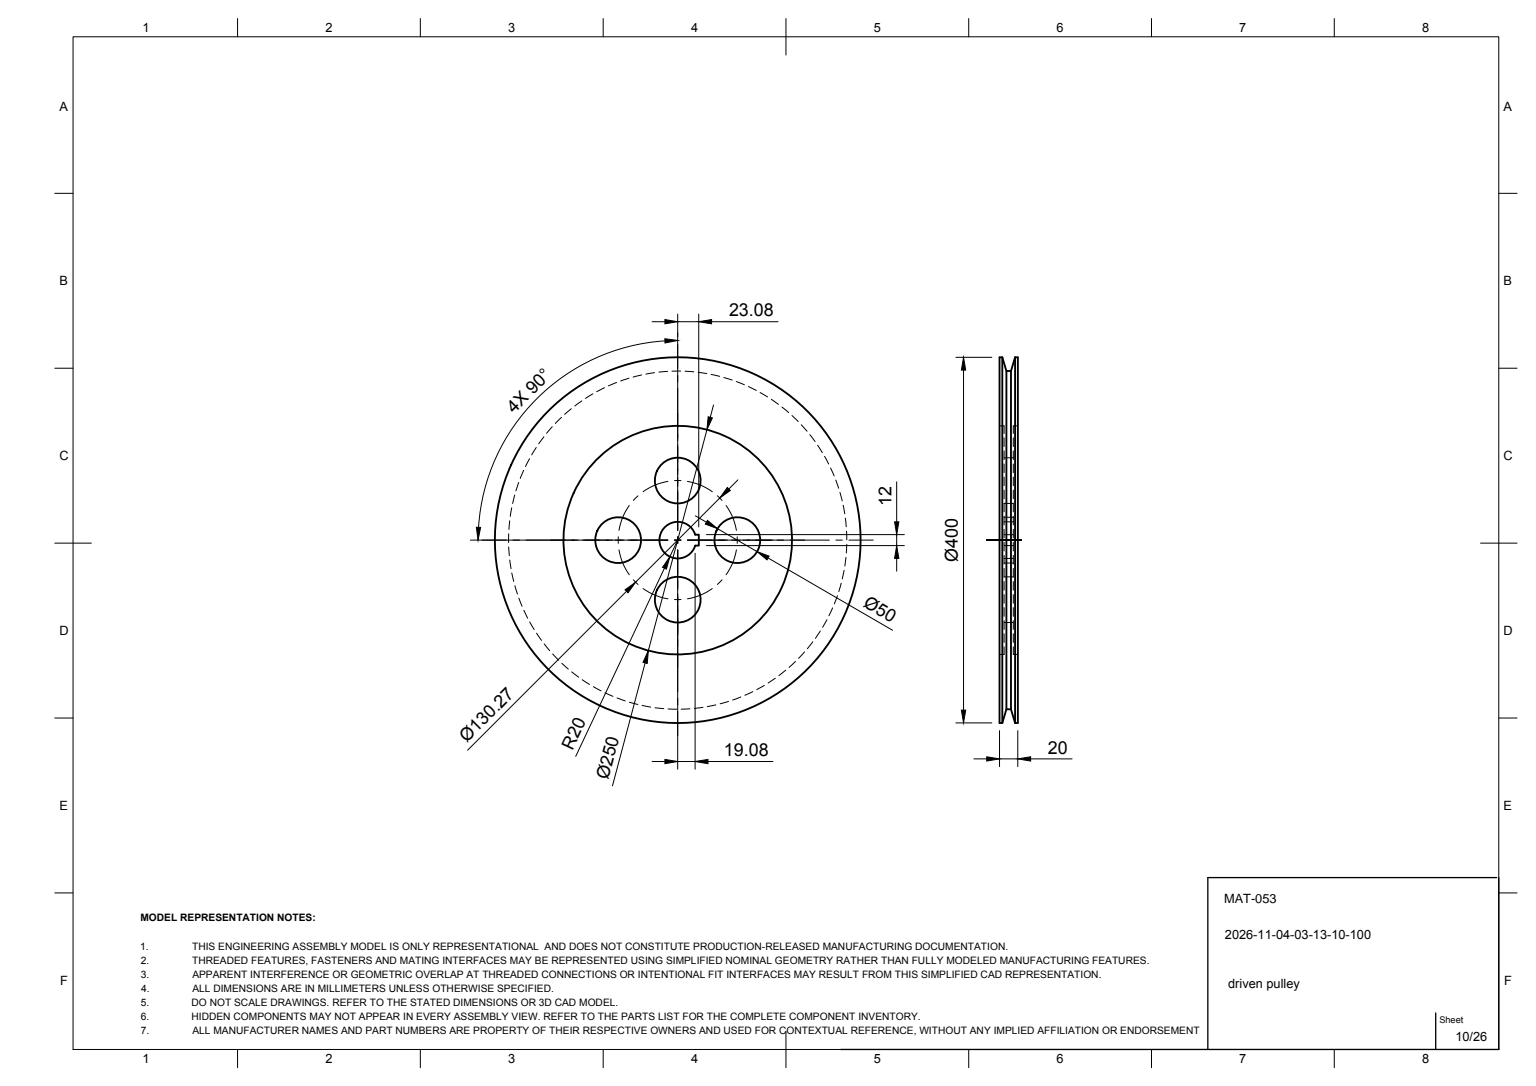
ISO-10303-21;
HEADER;
FILE_DESCRIPTION (('STEP AP214'),
    '1' );
FILE_NAME ('driven pulley.step',
    '2026-10-10T03:43:58',
    ( '' ),
    ( '' ),
    'SwSTEP 2.0',
    'SolidWorks 2026',
    '' );
FILE_SCHEMA (( 'AUTOMOTIVE_DESIGN' ));
ENDSEC;

DATA;
#14=EDGE_CURVE ( 'NONE', #39203, #23906, #5840, .T. ) ;
#73=PRODUCT_DEFINITION_CONTEXT ( 'detailed design', #24706, 'design' ) ;
#203=AXIS2_PLACEMENT_3D ( 'NONE', #23243, #1076, #59454 ) ;
#225=CARTESIAN_POINT ( 'NONE',  ( 90.13282190615606737, 1.839221433318906476E-12, 5.000000000000000000 ) ) ;
#267=CIRCLE ( 'NONE', #18213, 25.00000000000000000 ) ;
#269=ORIENTED_EDGE ( 'NONE', *, *, #50441, .F. ) ;
#325=CARTESIAN_POINT ( 'NONE',  ( 65.13282190615461786, 1.839221433318906476E-12, 5.000000000000000000 ) ) ;
#346=ORIENTED_EDGE ( 'NONE', *, *, #17053, .T. ) ;
#359=CARTESIAN_POINT ( 'NONE',  ( -65.13282190615095146, -1.847197903505587038E-12, 5.000000000000000000 ) ) ;
#383=VERTEX_POINT ( 'NONE', #55130 ) ;
#444=EDGE_LOOP ( 'NONE', ( #35988, #44492, #55517, #13641 ) ) ;
#462=AXIS2_PLACEMENT_3D ( 'NONE', #325, #22133, #54117 ) ;
#539=DIRECTION ( 'NONE',  ( 1.000000000000000000, 0.000000000000000000, 0.000000000000000000 ) ) ;
#586=ORIENTED_EDGE ( 'NONE', *, *, #6995, .F. ) ;
#619=AXIS2_PLACEMENT_3D ( 'NONE', #20593, #9026, #42056 ) ;
#711=CARTESIAN_POINT ( 'NONE',  ( 90.13282190615606737, 1.839221433318906476E-12, -5.000000000000000000 ) ) ;
#800=VECTOR ( 'NONE', #25987, 1000.000000000000000 ) ;
#856=EDGE_CURVE ( 'NONE', #15508, #55490, #4805, .T. ) ;
#868=DIRECTION ( 'NONE',  ( 0.000000000000000000, 1.000000000000000000, 0.000000000000000000 ) ) ;
#1003=VERTEX_POINT ( 'NONE', #17080 ) ;
#1034=DIRECTION ( 'NONE',  ( -1.000000000000000000, 0.000000000000000000, 0.000000000000000000 ) ) ;
#1076=DIRECTION ( 'NONE',  ( 0.000000000000000000, 0.000000000000000000, 1.000000000000000000 ) ) ;
#1234=AXIS2_PLACEMENT_3D ( 'NONE', #59286, #59624, #6531 ) ;
#1238=ORIENTED_EDGE ( 'NONE', *, *, #47800, .F. ) ;
#1338=EDGE_LOOP ( 'NONE', ( #14531, #35591, #15625, #48133 ) ) ;
#1340=CLOSED_SHELL ( 'NONE', ( #64564, #36434, #25846, #2769, #31042, #6717, #35413, #19813, #9481, #33980, #26616, #20112, #10478, #20014, #64798, #13207, #41216, #44725, #21120, #61014, #59716, #10226, #39239, #31844, #27146, #58887, #58375, #11492, #48120, #25762, #35077, #24104 ) ) ;
#1566=EDGE_LOOP ( 'NONE', ( #36926, #54120, #31121, #55593 ) ) ;
#1664=FACE_OUTER_BOUND ( 'NONE', #11943, .T. ) ;
#1697=DIRECTION ( 'NONE',  ( 0.000000000000000000, 0.000000000000000000, -1.000000000000000000 ) ) ;
#1938=VECTOR ( 'NONE', #46028, 1000.000000000000000 ) ;
#1973=DIRECTION ( 'NONE',  ( -0.000000000000000000, -0.000000000000000000, 1.000000000000000000 ) ) ;
#2092=ORIENTED_EDGE ( 'NONE', *, *, #5568, .T. ) ;
#2114=ORIENTED_EDGE ( 'NONE', *, *, #3365, .T. ) ;
#2123=EDGE_LOOP ( 'NONE', ( #65423, #20110, #20744, #32328 ) ) ;
#2127=ORIENTED_EDGE ( 'NONE', *, *, #52497, .F. ) ;
#2164=CARTESIAN_POINT ( 'NONE',  ( 0.000000000000000000, 0.000000000000000000, -5.000000000000000888 ) ) ;
#2182=EDGE_CURVE ( 'NONE', #46584, #55490, #14866, .T. ) ;
#2543=CIRCLE ( 'NONE', #21607, 25.00000000000395772 ) ;
#2575=EDGE_CURVE ( 'NONE', #49581, #11859, #45372, .T. ) ;
#2593=VERTEX_POINT ( 'NONE', #21779 ) ;
#2769=ADVANCED_FACE ( 'NONE', ( #66123 ), #11563, .F. ) ;
#2859=PLANE ( 'NONE',  #68017 ) ;
#3047=FACE_OUTER_BOUND ( 'NONE', #41666, .T. ) ;
#3053=AXIS2_PLACEMENT_3D ( 'NONE', #38989, #1697, #38628 ) ;
#3135=LINE ( 'NONE', #24596, #1938 ) ;
#3146=AXIS2_PLACEMENT_3D ( 'NONE', #50401, #40193, #18044 ) ;
#3280=EDGE_CURVE ( 'NONE', #66579, #13178, #38056, .T. ) ;
#3359=FACE_OUTER_BOUND ( 'NONE', #47238, .T. ) ;
#3365=EDGE_CURVE ( 'NONE', #383, #54841, #53079, .T. ) ;
#3381=DIRECTION ( 'NONE',  ( -0.000000000000000000, -0.000000000000000000, 1.000000000000000000 ) ) ;
#3395=DIRECTION ( 'NONE',  ( 1.000000000000000000, 0.000000000000000000, 0.000000000000000000 ) ) ;
#3412=DIRECTION ( 'NONE',  ( 0.000000000000000000, 0.000000000000000000, 1.000000000000000000 ) ) ;
#3472=SURFACE_SIDE_STYLE ('',( #51665 ) ) ;
#3504=DIRECTION ( 'NONE',  ( 1.000000000000000000, 0.000000000000000000, 0.000000000000000000 ) ) ;
#3630=AXIS2_PLACEMENT_3D ( 'NONE', #28129, #66490, #44673 ) ;
#3954=DIRECTION ( 'NONE',  ( 1.000000000000000000, 0.000000000000000000, 0.000000000000000000 ) ) ;
#3977=DIRECTION ( 'NONE',  ( -0.000000000000000000, -0.000000000000000000, 1.000000000000000000 ) ) ;
#4155=CARTESIAN_POINT ( 'NONE',  ( 0.000000000000000000, 65.13282190615278466, -5.000000000000000000 ) ) ;
#4242=CIRCLE ( 'NONE', #3146, 25.00000000000145306 ) ;
#4276=CIRCLE ( 'NONE', #68301, 25.00000000000296296 ) ;
#4368=DIRECTION ( 'NONE',  ( -0.000000000000000000, -0.000000000000000000, 1.000000000000000000 ) ) ;
#4663=CARTESIAN_POINT ( 'NONE',  ( 185.0000000000000000, 0.000000000000000000, 2.499999999999999556 ) ) ;
#4771=CARTESIAN_POINT ( 'NONE',  ( 0.000000000000000000, 0.000000000000000000, -10.00000000000000000 ) ) ;
#4792=AXIS2_PLACEMENT_3D ( 'NONE', #12377, #6038, #23634 ) ;
#4805=LINE ( 'NONE', #59305, #49723 ) ;
#4840=DIRECTION ( 'NONE',  ( 1.000000000000000000, 0.000000000000000000, 0.000000000000000000 ) ) ;
#4980=CIRCLE ( 'NONE', #462, 25.00000000000145306 ) ;
#5059=DIRECTION ( 'NONE',  ( -0.000000000000000000, -0.000000000000000000, 1.000000000000000000 ) ) ;
#5134=ORIENTED_EDGE ( 'NONE', *, *, #19397, .T. ) ;
#5201=DIRECTION ( 'NONE',  ( -0.000000000000000000, -0.000000000000000000, 1.000000000000000000 ) ) ;
#5272=CARTESIAN_POINT ( 'NONE',  ( -185.0000000000000000, 2.265596578422603396E-14, 2.499999999999999556 ) ) ;
#5548=SHAPE_REPRESENTATION ( 'driven pulley', ( #66832 ), #59007 ) ;
#5568=EDGE_CURVE ( 'NONE', #9677, #15508, #53224, .T. ) ;
#5588=LINE ( 'NONE', #59736, #24033 ) ;
#5840=CIRCLE ( 'NONE', #39560, 25.00000000000296296 ) ;
#5861=ORIENTED_EDGE ( 'NONE', *, *, #61188, .F. ) ;
#5890=DIRECTION ( 'NONE',  ( -1.000000000000000000, 0.000000000000000000, 0.000000000000000000 ) ) ;
#5975=CIRCLE ( 'NONE', #56554, 125.0000000000000000 ) ;
#5999=DIRECTION ( 'NONE',  ( 1.000000000000000000, 0.000000000000000000, 0.000000000000000000 ) ) ;
#6038=DIRECTION ( 'NONE',  ( -0.000000000000000000, -0.000000000000000000, 1.000000000000000000 ) ) ;
#6041=DIRECTION ( 'NONE',  ( 0.000000000000000000, 0.000000000000000000, -1.000000000000000000 ) ) ;
#6180=CARTESIAN_POINT ( 'NONE',  ( 0.000000000000000000, 0.000000000000000000, -10.00000000000000000 ) ) ;
#6277=CONICAL_SURFACE ( 'NONE', #41143, 185.0000000000000000, 1.279339532317029793 ) ;
#6321=PRODUCT ( 'driven pulley', 'driven pulley', '', ( #46640 ) ) ;
#6362=FACE_OUTER_BOUND ( 'NONE', #36222, .T. ) ;
#6459=CARTESIAN_POINT ( 'NONE',  ( 0.000000000000000000, 0.000000000000000000, -20.00000000000000000 ) ) ;
#6531=DIRECTION ( 'NONE',  ( 1.000000000000000000, 0.000000000000000000, 0.000000000000000000 ) ) ;
#6603=EDGE_CURVE ( 'NONE', #47682, #48865, #11766, .T. ) ;
#6627=ORIENTED_EDGE ( 'NONE', *, *, #14136, .F. ) ;
#6717=ADVANCED_FACE ( 'NONE', ( #19558 ), #41706, .F. ) ;
#6816=DIRECTION ( 'NONE',  ( -0.000000000000000000, -0.000000000000000000, 1.000000000000000000 ) ) ;
#6995=EDGE_CURVE ( 'NONE', #34341, #41500, #19660, .T. ) ;
#7019=VERTEX_POINT ( 'NONE', #14245 ) ;
#7023=EDGE_CURVE ( 'NONE', #8320, #22148, #29755, .T. ) ;
#7148=ORIENTED_EDGE ( 'NONE', *, *, #62973, .T. ) ;
#7149=VECTOR ( 'NONE', #29398, 1000.000000000000000 ) ;
#7158=CYLINDRICAL_SURFACE ( 'NONE', #45507, 25.00000000000000000 ) ;
#7185=ORIENTED_EDGE ( 'NONE', *, *, #60905, .F. ) ;
#7296=VECTOR ( 'NONE', #42362, 1000.000000000000000 ) ;
#7368=DIRECTION ( 'NONE',  ( -0.000000000000000000, -0.000000000000000000, 1.000000000000000000 ) ) ;
#7395=ORIENTED_EDGE ( 'NONE', *, *, #7023, .F. ) ;
#7432=EDGE_CURVE ( 'NONE', #19424, #25857, #61573, .T. ) ;
#7456=DIRECTION ( 'NONE',  ( -1.000000000000000000, 0.000000000000000000, 0.000000000000000000 ) ) ;
#7631=CARTESIAN_POINT ( 'NONE',  ( 200.0000000000000000, 2.449293598294706434E-14, -7.000000000000000000 ) ) ;
#7634=DIRECTION ( 'NONE',  ( 1.000000000000000000, 0.000000000000000000, -0.000000000000000000 ) ) ;
#7683=EDGE_LOOP ( 'NONE', ( #65023, #50621 ) ) ;
#7794=FACE_BOUND ( 'NONE', #49270, .T. ) ;
#7869=VECTOR ( 'NONE', #62960, 1000.000000000000000 ) ;
#7933=CYLINDRICAL_SURFACE ( 'NONE', #11850, 125.0000000000000000 ) ;
#7935=EDGE_CURVE ( 'NONE', #49581, #14060, #22990, .T. ) ;
#8124=CARTESIAN_POINT ( 'NONE',  ( 200.0000000000000000, 0.000000000000000000, -10.00000000000000000 ) ) ;
#8137=FACE_BOUND ( 'NONE', #65978, .T. ) ;
#8319=DIRECTION ( 'NONE',  ( 1.000000000000000000, 0.000000000000000000, 0.000000000000000000 ) ) ;
#8320=VERTEX_POINT ( 'NONE', #26711 ) ;
#8335=FACE_OUTER_BOUND ( 'NONE', #67692, .T. ) ;
#8424=AXIS2_PLACEMENT_3D ( 'NONE', #68725, #57497, #24461 ) ;
#8477=DIRECTION ( 'NONE',  ( 0.000000000000000000, 0.000000000000000000, -1.000000000000000000 ) ) ;
#8506=CARTESIAN_POINT ( 'NONE',  ( 0.000000000000000000, 0.000000000000000000, 5.000000000000000000 ) ) ;
#8766=FILL_AREA_STYLE ('',( #37197 ) ) ;
#8813=AXIS2_PLACEMENT_3D ( 'NONE', #50838, #35359, #24117 ) ;
#8817=FACE_OUTER_BOUND ( 'NONE', #68179, .T. ) ;
#9026=DIRECTION ( 'NONE',  ( -0.000000000000000000, -0.000000000000000000, 1.000000000000000000 ) ) ;
#9120=CIRCLE ( 'NONE', #67522, 200.0000000000000000 ) ;
#9344=ORIENTED_EDGE ( 'NONE', *, *, #14136, .T. ) ;
#9481=ADVANCED_FACE ( 'NONE', ( #55813 ), #57673, .F. ) ;
#9514=ORIENTED_EDGE ( 'NONE', *, *, #18668, .F. ) ;
#9516=CARTESIAN_POINT ( 'NONE',  ( 65.13282190615461786, 1.839221433318906476E-12, -5.000000000000000000 ) ) ;
#9594=DIRECTION ( 'NONE',  ( 1.000000000000000000, 0.000000000000000000, 0.000000000000000000 ) ) ;
#9605=EDGE_CURVE ( 'NONE', #11859, #49581, #63695, .T. ) ;
#9650=ORIENTED_EDGE ( 'NONE', *, *, #43482, .T. ) ;
#9656=DIRECTION ( 'NONE',  ( -0.000000000000000000, -0.000000000000000000, 1.000000000000000000 ) ) ;
#9662=CIRCLE ( 'NONE', #62435, 25.00000000000000000 ) ;
#9677=VERTEX_POINT ( 'NONE', #40367 ) ;
#9720=DIRECTION ( 'NONE',  ( 1.000000000000000000, 0.000000000000000000, 0.000000000000000000 ) ) ;
#9736=ORIENTED_EDGE ( 'NONE', *, *, #9605, .T. ) ;
#9853=VECTOR ( 'NONE', #9873, 1000.000000000000227 ) ;
#9873=DIRECTION ( 'NONE',  ( -0.9578262852211514300, 1.172998894335282758E-16, 0.2873478855663451625 ) ) ;
#9903=ORIENTED_EDGE ( 'NONE', *, *, #60097, .T. ) ;
#9908=CIRCLE ( 'NONE', #8813, 125.0000000000000000 ) ;
#9932=ORIENTED_EDGE ( 'NONE', *, *, #24558, .T. ) ;
#10055=CYLINDRICAL_SURFACE ( 'NONE', #17941, 200.0000000000000000 ) ;
#10121=DIRECTION ( 'NONE',  ( -0.000000000000000000, -0.000000000000000000, 1.000000000000000000 ) ) ;
#10127=VECTOR ( 'NONE', #6816, 1000.000000000000000 ) ;
#10174=LINE ( 'NONE', #15801, #50169 ) ;
#10226=ADVANCED_FACE ( 'NONE', ( #11029 ), #47964, .F. ) ;
#10305=DIRECTION ( 'NONE',  ( 1.000000000000000000, 0.000000000000000000, 0.000000000000000000 ) ) ;
#10478=ADVANCED_FACE ( 'NONE', ( #14503 ), #52136, .T. ) ;
#10651=VECTOR ( 'NONE', #35516, 1000.000000000000000 ) ;
#10757=VECTOR ( 'NONE', #66610, 1000.000000000000000 ) ;
#10776=FACE_OUTER_BOUND ( 'NONE', #60970, .T. ) ;
#10963=DIRECTION ( 'NONE',  ( 1.000000000000000000, 0.000000000000000000, 0.000000000000000000 ) ) ;
#11029=FACE_OUTER_BOUND ( 'NONE', #32271, .T. ) ;
#11237=EDGE_LOOP ( 'NONE', ( #63243, #586 ) ) ;
#11388=ORIENTED_EDGE ( 'NONE', *, *, #22251, .T. ) ;
#11419=CARTESIAN_POINT ( 'NONE',  ( 0.000000000000000000, 0.000000000000000000, 7.000000000000000000 ) ) ;
#11460=DIRECTION ( 'NONE',  ( -0.000000000000000000, -0.000000000000000000, 1.000000000000000000 ) ) ;
#11492=ADVANCED_FACE ( 'NONE', ( #63054 ), #36325, .T. ) ;
#11563=CYLINDRICAL_SURFACE ( 'NONE', #66742, 25.00000000000000000 ) ;
#11570=EDGE_CURVE ( 'NONE', #48842, #30587, #49206, .T. ) ;
#11594=DIRECTION ( 'NONE',  ( 1.000000000000000000, 0.000000000000000000, 0.000000000000000000 ) ) ;
#11613=FACE_OUTER_BOUND ( 'NONE', #444, .T. ) ;
#11727=DIRECTION ( 'NONE',  ( 1.000000000000000000, 0.000000000000000000, 0.000000000000000000 ) ) ;
#11754=DIRECTION ( 'NONE',  ( 0.000000000000000000, 0.000000000000000000, -1.000000000000000000 ) ) ;
#11766=CIRCLE ( 'NONE', #51098, 25.00000000000395772 ) ;
#11847=DIRECTION ( 'NONE',  ( 0.000000000000000000, 0.000000000000000000, 1.000000000000000000 ) ) ;
#11850=AXIS2_PLACEMENT_3D ( 'NONE', #55413, #1973, #39938 ) ;
#11859=VERTEX_POINT ( 'NONE', #41177 ) ;
#11943=EDGE_LOOP ( 'NONE', ( #55108, #57726, #64257, #269 ) ) ;
#12116=UNCERTAINTY_MEASURE_WITH_UNIT (LENGTH_MEASURE( 1.000000000000000082E-05 ), #53269, 'distance_accuracy_value', 'NONE');
#12144=EDGE_CURVE ( 'NONE', #41500, #34341, #36731, .T. ) ;
#12358=CARTESIAN_POINT ( 'NONE',  ( -40.13282190614798850, -1.847197903505587038E-12, -9.999999999999998224 ) ) ;
#12377=CARTESIAN_POINT ( 'NONE',  ( 0.000000000000000000, 0.000000000000000000, -2.500000000000002220 ) ) ;
#12449=LINE ( 'NONE', #22649, #10127 ) ;
#12453=VERTEX_POINT ( 'NONE', #39536 ) ;
#12555=DIRECTION ( 'NONE',  ( 1.000000000000000000, 0.000000000000000000, 0.000000000000000000 ) ) ;
#12588=( GEOMETRIC_REPRESENTATION_CONTEXT ( 3 ) GLOBAL_UNCERTAINTY_ASSIGNED_CONTEXT ( ( #66299 ) ) GLOBAL_UNIT_ASSIGNED_CONTEXT ( ( #52001, #41456, #58642 ) ) REPRESENTATION_CONTEXT ( 'NONE', 'WORKASPACE' ) );
#12731=DIRECTION ( 'NONE',  ( 0.000000000000000000, 0.000000000000000000, -1.000000000000000000 ) ) ;
#12848=CARTESIAN_POINT ( 'NONE',  ( -6.000000000000000000, 23.07878402833891229, -5.000000000000000000 ) ) ;
#12948=AXIS2_PLACEMENT_3D ( 'NONE', #36428, #57883, #43795 ) ;
#13029=AXIS2_PLACEMENT_3D ( 'NONE', #6180, #59296, #49077 ) ;
#13063=EDGE_LOOP ( 'NONE', ( #44716, #16709 ) ) ;
#13178=VERTEX_POINT ( 'NONE', #62526 ) ;
#13207=ADVANCED_FACE ( 'NONE', ( #46681, #13987 ), #13638, .F. ) ;
#13252=ORIENTED_EDGE ( 'NONE', *, *, #49764, .T. ) ;
#13260=EDGE_CURVE ( 'NONE', #46584, #50826, #36135, .T. ) ;
#13273=EDGE_CURVE ( 'NONE', #2593, #1003, #15018, .T. ) ;
#13280=AXIS2_PLACEMENT_3D ( 'NONE', #24520, #61100, #3395 ) ;
#13357=CARTESIAN_POINT ( 'NONE',  ( 3.678442866637813759E-12, -65.13282190615278466, -9.999999999999998224 ) ) ;
#13638=PLANE ( 'NONE',  #57238 ) ;
#13640=EDGE_LOOP ( 'NONE', ( #55151, #346, #49689, #9903 ) ) ;
#13641=ORIENTED_EDGE ( 'NONE', *, *, #27798, .F. ) ;
#13927=AXIS2_PLACEMENT_3D ( 'NONE', #54921, #65496, #7456 ) ;
#13987=FACE_OUTER_BOUND ( 'NONE', #47331, .T. ) ;
#14003=VERTEX_POINT ( 'NONE', #63226 ) ;
#14004=LINE ( 'NONE', #25264, #36379 ) ;
#14006=ORIENTED_EDGE ( 'NONE', *, *, #50811, .F. ) ;
#14029=DIRECTION ( 'NONE',  ( -0.000000000000000000, -0.000000000000000000, 1.000000000000000000 ) ) ;
#14054=CARTESIAN_POINT ( 'NONE',  ( 40.13282190615316836, 1.842283050316774879E-12, -9.999999999999998224 ) ) ;
#14060=VERTEX_POINT ( 'NONE', #225 ) ;
#14136=EDGE_CURVE ( 'NONE', #49232, #40260, #32255, .T. ) ;
#14160=ORIENTED_EDGE ( 'NONE', *, *, #45668, .T. ) ;
#14176=ORIENTED_EDGE ( 'NONE', *, *, #12144, .T. ) ;
#14245=CARTESIAN_POINT ( 'NONE',  ( -125.0000000000000000, 1.530808498934191561E-14, 10.00000000000000000 ) ) ;
#14436=LINE ( 'NONE', #35886, #7869 ) ;
#14503=FACE_OUTER_BOUND ( 'NONE', #42414, .T. ) ;
#14531=ORIENTED_EDGE ( 'NONE', *, *, #48902, .T. ) ;
#14558=EDGE_CURVE ( 'NONE', #22538, #40260, #28097, .T. ) ;
#14562=ORIENTED_EDGE ( 'NONE', *, *, #64384, .T. ) ;
#14594=LINE ( 'NONE', #57510, #7296 ) ;
#14599=DIRECTION ( 'NONE',  ( 1.000000000000000000, 0.000000000000000000, 0.000000000000000000 ) ) ;
#14636=EDGE_CURVE ( 'NONE', #22148, #7019, #12449, .T. ) ;
#14671=CARTESIAN_POINT ( 'NONE',  ( 0.000000000000000000, 0.000000000000000000, -10.00000000000000000 ) ) ;
#14693=CARTESIAN_POINT ( 'NONE',  ( -125.0000000000000000, 1.530808498934191561E-14, 5.000000000000000000 ) ) ;
#14839=FACE_OUTER_BOUND ( 'NONE', #54551, .T. ) ;
#14866=LINE ( 'NONE', #15907, #32968 ) ;
#15018=LINE ( 'NONE', #36481, #51616 ) ;
#15085=VECTOR ( 'NONE', #7368, 1000.000000000000000 ) ;
#15127=VERTEX_POINT ( 'NONE', #54034 ) ;
#15371=AXIS2_PLACEMENT_3D ( 'NONE', #21361, #10121, #4840 ) ;
#15442=AXIS2_PLACEMENT_3D ( 'NONE', #6459, #5059, #17347 ) ;
#15508=VERTEX_POINT ( 'NONE', #34629 ) ;
#15539=CARTESIAN_POINT ( 'NONE',  ( 0.000000000000000000, 0.000000000000000000, 7.000000000000000000 ) ) ;
#15543=CARTESIAN_POINT ( 'NONE',  ( -25.00000000000000000, 65.13282190615278466, -5.000000000000000000 ) ) ;
#15625=ORIENTED_EDGE ( 'NONE', *, *, #55396, .T. ) ;
#15739=VERTEX_POINT ( 'NONE', #15543 ) ;
#15801=CARTESIAN_POINT ( 'NONE',  ( 6.000000000000000000, 0.000000000000000000, 5.000000000000000000 ) ) ;
#15907=CARTESIAN_POINT ( 'NONE',  ( -6.000000000000000000, 23.07878402833891229, 9.999999999999998224 ) ) ;
#15924=EDGE_LOOP ( 'NONE', ( #27771, #58045 ) ) ;
#16004=SHAPE_DEFINITION_REPRESENTATION ( #22614, #5548 ) ;
#16034=VECTOR ( 'NONE', #26129, 1000.000000000000227 ) ;
#16044=ORIENTED_EDGE ( 'NONE', *, *, #22064, .F. ) ;
#16128=DIRECTION ( 'NONE',  ( -0.000000000000000000, -0.000000000000000000, 1.000000000000000000 ) ) ;
#16129=CIRCLE ( 'NONE', #37463, 185.0000000000000000 ) ;
#16199=VERTEX_POINT ( 'NONE', #19533 ) ;
#16296=CARTESIAN_POINT ( 'NONE',  ( 0.000000000000000000, 0.000000000000000000, 2.499999999999999556 ) ) ;
#16353=ORIENTED_EDGE ( 'NONE', *, *, #27798, .T. ) ;
#16367=CIRCLE ( 'NONE', #13029, 200.0000000000000000 ) ;
#16554=CIRCLE ( 'NONE', #34567, 20.00000000000000000 ) ;
#16564=CARTESIAN_POINT ( 'NONE',  ( 6.000000000000000000, 23.07878402833891229, 9.999999999999998224 ) ) ;
#16610=CONICAL_SURFACE ( 'NONE', #40229, 200.0000000000000000, 1.279339532317029793 ) ;
#16709=ORIENTED_EDGE ( 'NONE', *, *, #9605, .F. ) ;
#16880=AXIS2_PLACEMENT_3D ( 'NONE', #67142, #46691, #50938 ) ;
#16906=DIRECTION ( 'NONE',  ( -0.000000000000000000, -0.000000000000000000, -1.000000000000000000 ) ) ;
#16915=CARTESIAN_POINT ( 'NONE',  ( 200.0000000000000000, 0.000000000000000000, -7.000000000000000000 ) ) ;
#17022=SHAPE_REPRESENTATION_RELATIONSHIP ( 'NONE' , 'NONE' ,  #5548, #33268 ) ;
#17053=EDGE_CURVE ( 'NONE', #15739, #2593, #267, .T. ) ;
#17080=CARTESIAN_POINT ( 'NONE',  ( 25.00000000000000000, 65.13282190615278466, 5.000000000000000000 ) ) ;
#17159=CARTESIAN_POINT ( 'NONE',  ( 125.0000000000000000, 1.530808498934191561E-14, -5.000000000000000000 ) ) ;
#17347=DIRECTION ( 'NONE',  ( 1.000000000000000000, 0.000000000000000000, 0.000000000000000000 ) ) ;
#17397=LINE ( 'NONE', #60663, #62487 ) ;
#17536=CIRCLE ( 'NONE', #48948, 200.0000000000000000 ) ;
#17603=FACE_OUTER_BOUND ( 'NONE', #19671, .T. ) ;
#17649=ORIENTED_EDGE ( 'NONE', *, *, #57077, .T. ) ;
#17689=AXIS2_PLACEMENT_3D ( 'NONE', #48586, #6041, #63769 ) ;
#17734=DIRECTION ( 'NONE',  ( 0.000000000000000000, 0.000000000000000000, 1.000000000000000000 ) ) ;
#17736=ORIENTED_EDGE ( 'NONE', *, *, #14636, .T. ) ;
#17922=MANIFOLD_SOLID_BREP ( 'Cut-Extrude4', #1340 ) ;
#17941=AXIS2_PLACEMENT_3D ( 'NONE', #4771, #42409, #9720 ) ;
#18044=DIRECTION ( 'NONE',  ( 1.000000000000000000, 0.000000000000000000, 0.000000000000000000 ) ) ;
#18087=CARTESIAN_POINT ( 'NONE',  ( -20.00000000000000000, 2.449293598294706513E-15, 5.000000000000000000 ) ) ;
#18163=ORIENTED_EDGE ( 'NONE', *, *, #13260, .F. ) ;
#18205=AXIS2_PLACEMENT_3D ( 'NONE', #28227, #39156, #54964 ) ;
#18213=AXIS2_PLACEMENT_3D ( 'NONE', #4155, #20663, #67832 ) ;
#18273=CARTESIAN_POINT ( 'NONE',  ( -185.0000000000000000, 2.265596578422603396E-14, 0.000000000000000000 ) ) ;
#18483=ORIENTED_EDGE ( 'NONE', *, *, #14, .F. ) ;
#18581=DIRECTION ( 'NONE',  ( -1.000000000000000000, 0.000000000000000000, 0.000000000000000000 ) ) ;
#18626=FACE_OUTER_BOUND ( 'NONE', #24803, .T. ) ;
#18668=EDGE_CURVE ( 'NONE', #13178, #61651, #9120, .T. ) ;
#18759=AXIS2_PLACEMENT_3D ( 'NONE', #21403, #16128, #37584 ) ;
#18905=EDGE_CURVE ( 'NONE', #22148, #8320, #60773, .T. ) ;
#19110=EDGE_LOOP ( 'NONE', ( #44365, #56046 ) ) ;
#19149=ORIENTED_EDGE ( 'NONE', *, *, #856, .T. ) ;
#19201=PLANE ( 'NONE',  #59888 ) ;
#19209=CIRCLE ( 'NONE', #1234, 200.0000000000000000 ) ;
#19217=DIRECTION ( 'NONE',  ( -1.000000000000000000, 0.000000000000000000, 0.000000000000000000 ) ) ;
#19225=ORIENTED_EDGE ( 'NONE', *, *, #60905, .T. ) ;
#19352=AXIS2_PLACEMENT_3D ( 'NONE', #39406, #38355, #60854 ) ;
#19397=EDGE_CURVE ( 'NONE', #40260, #19424, #46211, .T. ) ;
#19424=VERTEX_POINT ( 'NONE', #24872 ) ;
#19500=AXIS2_PLACEMENT_3D ( 'NONE', #36849, #46702, #62891 ) ;
#19533=CARTESIAN_POINT ( 'NONE',  ( -200.0000000000000000, 2.449293598294706434E-14, -7.000000000000000000 ) ) ;
#19558=FACE_OUTER_BOUND ( 'NONE', #2123, .T. ) ;
#19571=CYLINDRICAL_SURFACE ( 'NONE', #42294, 125.0000000000000000 ) ;
#19645=PRESENTATION_STYLE_ASSIGNMENT (( #24933 ) ) ;
#19655=AXIS2_PLACEMENT_3D ( 'NONE', #53954, #868, #32190 ) ;
#19660=CIRCLE ( 'NONE', #42097, 125.0000000000000000 ) ;
#19671=EDGE_LOOP ( 'NONE', ( #37736, #47416, #9650, #43541 ) ) ;
#19699=CIRCLE ( 'NONE', #35423, 125.0000000000000000 ) ;
#19813=ADVANCED_FACE ( 'NONE', ( #50398 ), #50045, .F. ) ;
#19817=AXIS2_PLACEMENT_3D ( 'NONE', #58441, #37333, #32071 ) ;
#20009=CARTESIAN_POINT ( 'NONE',  ( 125.0000000000000000, 0.000000000000000000, 5.000000000000000000 ) ) ;
#20014=ADVANCED_FACE ( 'NONE', ( #17603 ), #48533, .T. ) ;
#20076=DIRECTION ( 'NONE',  ( 0.000000000000000000, 0.000000000000000000, -1.000000000000000000 ) ) ;
#20110=ORIENTED_EDGE ( 'NONE', *, *, #35090, .T. ) ;
#20112=ADVANCED_FACE ( 'NONE', ( #11613 ), #55225, .T. ) ;
#20210=ORIENTED_EDGE ( 'NONE', *, *, #67936, .T. ) ;
#20221=DIRECTION ( 'NONE',  ( -0.000000000000000000, -0.000000000000000000, 1.000000000000000000 ) ) ;
#20277=ORIENTED_EDGE ( 'NONE', *, *, #18668, .T. ) ;
#20402=AXIS2_PLACEMENT_3D ( 'NONE', #62507, #3412, #40349 ) ;
#20454=CIRCLE ( 'NONE', #50796, 200.0000000000000000 ) ;
#20459=CYLINDRICAL_SURFACE ( 'NONE', #44391, 125.0000000000000000 ) ;
#20508=DIRECTION ( 'NONE',  ( -0.000000000000000000, -0.000000000000000000, 1.000000000000000000 ) ) ;
#20593=CARTESIAN_POINT ( 'NONE',  ( 0.000000000000000000, 0.000000000000000000, -7.000000000000000000 ) ) ;
#20663=DIRECTION ( 'NONE',  ( 0.000000000000000000, 0.000000000000000000, -1.000000000000000000 ) ) ;
#20681=ORIENTED_EDGE ( 'NONE', *, *, #66289, .T. ) ;
#20744=ORIENTED_EDGE ( 'NONE', *, *, #6603, .T. ) ;
#20831=CARTESIAN_POINT ( 'NONE',  ( 0.000000000000000000, 0.000000000000000000, 0.000000000000000000 ) ) ;
#20906=VECTOR ( 'NONE', #16906, 1000.000000000000000 ) ;
#20924=ORIENTED_EDGE ( 'NONE', *, *, #48453, .T. ) ;
#21120=ADVANCED_FACE ( 'NONE', ( #41765, #62877, #47366, #31221, #46688, #56912 ), #57938, .T. ) ;
#21361=CARTESIAN_POINT ( 'NONE',  ( 0.000000000000000000, 0.000000000000000000, 2.499999999999999556 ) ) ;
#21390=ORIENTED_EDGE ( 'NONE', *, *, #58327, .T. ) ;
#21403=CARTESIAN_POINT ( 'NONE',  ( 0.000000000000000000, 0.000000000000000000, -20.00000000000000000 ) ) ;
#21607=AXIS2_PLACEMENT_3D ( 'NONE', #23866, #66793, #18581 ) ;
#21663=EDGE_CURVE ( 'NONE', #9677, #22538, #57861, .T. ) ;
#21760=DIRECTION ( 'NONE',  ( -0.000000000000000000, 1.000000000000000000, 0.000000000000000000 ) ) ;
#21767=DIRECTION ( 'NONE',  ( -0.000000000000000000, -0.000000000000000000, 1.000000000000000000 ) ) ;
#21779=CARTESIAN_POINT ( 'NONE',  ( 25.00000000000000000, 65.13282190615278466, -5.000000000000000000 ) ) ;
#22006=ORIENTED_EDGE ( 'NONE', *, *, #29771, .F. ) ;
#22064=EDGE_CURVE ( 'NONE', #48865, #47682, #49816, .T. ) ;
#22133=DIRECTION ( 'NONE',  ( 0.000000000000000000, 0.000000000000000000, 1.000000000000000000 ) ) ;
#22135=ORIENTED_EDGE ( 'NONE', *, *, #45668, .F. ) ;
#22148=VERTEX_POINT ( 'NONE', #14693 ) ;
#22169=PLANE ( 'NONE',  #56871 ) ;
#22194=LINE ( 'NONE', #16564, #20906 ) ;
#22251=EDGE_CURVE ( 'NONE', #7019, #15127, #5975, .T. ) ;
#22360=VERTEX_POINT ( 'NONE', #49810 ) ;
#22391=DIRECTION ( 'NONE',  ( 1.000000000000000000, 0.000000000000000000, 0.000000000000000000 ) ) ;
#22538=VERTEX_POINT ( 'NONE', #18087 ) ;
#22614=PRODUCT_DEFINITION_SHAPE ( 'NONE', 'NONE',  #63276 ) ;
#22649=CARTESIAN_POINT ( 'NONE',  ( -125.0000000000000000, 1.530808498934191561E-14, 5.000000000000000000 ) ) ;
#22852=EDGE_CURVE ( 'NONE', #2593, #15739, #39742, .T. ) ;
#22990=LINE ( 'NONE', #44434, #10757 ) ;
#23128=AXIS2_PLACEMENT_3D ( 'NONE', #27817, #28518, #5999 ) ;
#23243=CARTESIAN_POINT ( 'NONE',  ( 0.000000000000000000, 0.000000000000000000, -10.00000000000000000 ) ) ;
#23277=CARTESIAN_POINT ( 'NONE',  ( -6.000000000000000000, 23.07878402833891229, 5.000000000000000000 ) ) ;
#23281=AXIS2_PLACEMENT_3D ( 'NONE', #49898, #60100, #66457 ) ;
#23352=FACE_OUTER_BOUND ( 'NONE', #13640, .T. ) ;
#23463=DIRECTION ( 'NONE',  ( 1.000000000000000000, 0.000000000000000000, 0.000000000000000000 ) ) ;
#23529=EDGE_LOOP ( 'NONE', ( #32810, #33867, #50728, #28320 ) ) ;
#23557=DIRECTION ( 'NONE',  ( -0.000000000000000000, -0.000000000000000000, 1.000000000000000000 ) ) ;
#23613=VERTEX_POINT ( 'NONE', #55185 ) ;
#23634=DIRECTION ( 'NONE',  ( 1.000000000000000000, 0.000000000000000000, 0.000000000000000000 ) ) ;
#23699=EDGE_CURVE ( 'NONE', #383, #66579, #40401, .T. ) ;
#23781=CARTESIAN_POINT ( 'NONE',  ( -185.0000000000000000, 2.357445088358655073E-14, 2.499999999999999556 ) ) ;
#23816=CYLINDRICAL_SURFACE ( 'NONE', #13280, 25.00000000000145306 ) ;
#23828=ORIENTED_EDGE ( 'NONE', *, *, #52622, .T. ) ;
#23866=CARTESIAN_POINT ( 'NONE',  ( 3.678442866637813759E-12, -65.13282190615278466, -5.000000000000000000 ) ) ;
#23906=VERTEX_POINT ( 'NONE', #69540 ) ;
#24033=VECTOR ( 'NONE', #21767, 1000.000000000000000 ) ;
#24104=ADVANCED_FACE ( 'NONE', ( #37446 ), #47656, .F. ) ;
#24117=DIRECTION ( 'NONE',  ( 1.000000000000000000, 0.000000000000000000, 0.000000000000000000 ) ) ;
#24429=ORIENTED_EDGE ( 'NONE', *, *, #38176, .F. ) ;
#24461=DIRECTION ( 'NONE',  ( 1.000000000000000000, 0.000000000000000000, 0.000000000000000000 ) ) ;
#24508=CARTESIAN_POINT ( 'NONE',  ( 0.000000000000000000, 0.000000000000000000, 10.00000000000000000 ) ) ;
#24520=CARTESIAN_POINT ( 'NONE',  ( 65.13282190615461786, 1.839221433318906476E-12, -9.999999999999998224 ) ) ;
#24558=EDGE_CURVE ( 'NONE', #15127, #7019, #19699, .T. ) ;
#24596=CARTESIAN_POINT ( 'NONE',  ( -125.0000000000000000, 0.000000000000000000, -5.000000000000000000 ) ) ;
#24706=APPLICATION_CONTEXT ( 'automotive_design' ) ;
#24755=AXIS2_PLACEMENT_3D ( 'NONE', #33572, #17734, #66622 ) ;
#24803=EDGE_LOOP ( 'NONE', ( #53971, #23828, #40146, #57589 ) ) ;
#24805=EDGE_CURVE ( 'NONE', #34775, #16199, #44397, .T. ) ;
#24817=CYLINDRICAL_SURFACE ( 'NONE', #29795, 25.00000000000145306 ) ;
#24872=CARTESIAN_POINT ( 'NONE',  ( 6.000000000000000000, 19.07878402833891229, 4.999999999999997335 ) ) ;
#24933=SURFACE_STYLE_USAGE ( .BOTH. , #3472 ) ;
#24969=ORIENTED_EDGE ( 'NONE', *, *, #7023, .T. ) ;
#25213=FACE_OUTER_BOUND ( 'NONE', #43198, .T. ) ;
#25215=ORIENTED_EDGE ( 'NONE', *, *, #59128, .T. ) ;
#25255=CYLINDRICAL_SURFACE ( 'NONE', #16880, 25.00000000000296296 ) ;
#25264=CARTESIAN_POINT ( 'NONE',  ( -200.0000000000000000, 2.449293598294706434E-14, -10.00000000000000000 ) ) ;
#25296=ORIENTED_EDGE ( 'NONE', *, *, #29875, .F. ) ;
#25762=ADVANCED_FACE ( 'NONE', ( #27432 ), #22169, .F. ) ;
#25808=LINE ( 'NONE', #69393, #58241 ) ;
#25846=ADVANCED_FACE ( 'NONE', ( #38698 ), #6277, .T. ) ;
#25857=VERTEX_POINT ( 'NONE', #33075 ) ;
#25987=DIRECTION ( 'NONE',  ( 0.000000000000000000, -1.000000000000000000, 0.000000000000000000 ) ) ;
#26076=ORIENTED_EDGE ( 'NONE', *, *, #44634, .F. ) ;
#26129=DIRECTION ( 'NONE',  ( 0.9578262852211514300, 0.000000000000000000, 0.2873478855663451625 ) ) ;
#26151=ORIENTED_EDGE ( 'NONE', *, *, #17053, .F. ) ;
#26153=CARTESIAN_POINT ( 'NONE',  ( 0.000000000000000000, 0.000000000000000000, 5.000000000000000000 ) ) ;
#26405=CARTESIAN_POINT ( 'NONE',  ( -40.13282190614798850, -1.847197903505587038E-12, -5.000000000000000000 ) ) ;
#26437=DIRECTION ( 'NONE',  ( -0.000000000000000000, -0.000000000000000000, -1.000000000000000000 ) ) ;
#26576=VECTOR ( 'NONE', #59651, 1000.000000000000000 ) ;
#26616=ADVANCED_FACE ( 'NONE', ( #14839 ), #20459, .F. ) ;
#26711=CARTESIAN_POINT ( 'NONE',  ( 125.0000000000000000, 0.000000000000000000, 5.000000000000000000 ) ) ;
#26713=VECTOR ( 'NONE', #23557, 1000.000000000000000 ) ;
#26852=DIRECTION ( 'NONE',  ( 1.000000000000000000, 0.000000000000000000, 0.000000000000000000 ) ) ;
#26896=CARTESIAN_POINT ( 'NONE',  ( -65.13282190615095146, -1.847197903505587038E-12, -5.000000000000000000 ) ) ;
#26898=( NAMED_UNIT ( * ) SI_UNIT ( $, .STERADIAN. ) SOLID_ANGLE_UNIT ( ) );
#27043=ORIENTED_EDGE ( 'NONE', *, *, #57077, .F. ) ;
#27146=ADVANCED_FACE ( 'NONE', ( #3359 ), #24817, .F. ) ;
#27213=VERTEX_POINT ( 'NONE', #53934 ) ;
#27225=ORIENTED_EDGE ( 'NONE', *, *, #30249, .F. ) ;
#27227=AXIS2_PLACEMENT_3D ( 'NONE', #50247, #29480, #44620 ) ;
#27297=DIRECTION ( 'NONE',  ( 1.000000000000000000, 0.000000000000000000, 0.000000000000000000 ) ) ;
#27353=EDGE_LOOP ( 'NONE', ( #2114, #20924, #45858, #54114 ) ) ;
#27432=FACE_OUTER_BOUND ( 'NONE', #42884, .T. ) ;
#27653=CARTESIAN_POINT ( 'NONE',  ( 20.00000000000000000, 0.000000000000000000, -20.00000000000000000 ) ) ;
#27751=EDGE_CURVE ( 'NONE', #49232, #9677, #48879, .T. ) ;
#27771=ORIENTED_EDGE ( 'NONE', *, *, #63600, .T. ) ;
#27798=EDGE_CURVE ( 'NONE', #22360, #34775, #29236, .T. ) ;
#27817=CARTESIAN_POINT ( 'NONE',  ( 0.000000000000000000, 0.000000000000000000, 2.499999999999999556 ) ) ;
#27839=DIRECTION ( 'NONE',  ( -0.000000000000000000, -0.000000000000000000, 1.000000000000000000 ) ) ;
#28061=ORIENTED_EDGE ( 'NONE', *, *, #14636, .F. ) ;
#28097=CIRCLE ( 'NONE', #24755, 20.00000000000000000 ) ;
#28129=CARTESIAN_POINT ( 'NONE',  ( -65.13282190615095146, -1.847197903505587038E-12, -5.000000000000000000 ) ) ;
#28227=CARTESIAN_POINT ( 'NONE',  ( 0.000000000000000000, 0.000000000000000000, -20.00000000000000000 ) ) ;
#28320=ORIENTED_EDGE ( 'NONE', *, *, #39557, .F. ) ;
#28335=FACE_OUTER_BOUND ( 'NONE', #45849, .T. ) ;
#28388=CARTESIAN_POINT ( 'NONE',  ( 25.00000000000763478, -65.13282190615278466, 5.000000000000000000 ) ) ;
#28518=DIRECTION ( 'NONE',  ( -0.000000000000000000, -0.000000000000000000, 1.000000000000000000 ) ) ;
#28792=VECTOR ( 'NONE', #14029, 1000.000000000000000 ) ;
#29045=AXIS2_PLACEMENT_3D ( 'NONE', #45000, #34476, #44670 ) ;
#29236=LINE ( 'NONE', #8124, #64633 ) ;
#29257=DIRECTION ( 'NONE',  ( -1.000000000000000000, 0.000000000000000000, 0.000000000000000000 ) ) ;
#29280=VERTEX_POINT ( 'NONE', #37196 ) ;
#29398=DIRECTION ( 'NONE',  ( -0.000000000000000000, -0.000000000000000000, 1.000000000000000000 ) ) ;
#29443=CIRCLE ( 'NONE', #3630, 25.00000000000296296 ) ;
#29480=DIRECTION ( 'NONE',  ( -0.000000000000000000, -0.000000000000000000, 1.000000000000000000 ) ) ;
#29571=DIRECTION ( 'NONE',  ( 0.000000000000000000, 0.000000000000000000, 1.000000000000000000 ) ) ;
#29580=FACE_BOUND ( 'NONE', #54135, .T. ) ;
#29723=DIRECTION ( 'NONE',  ( 1.000000000000000000, 0.000000000000000000, 0.000000000000000000 ) ) ;
#29755=CIRCLE ( 'NONE', #8424, 125.0000000000000000 ) ;
#29771=EDGE_CURVE ( 'NONE', #41500, #30587, #3135, .T. ) ;
#29795=AXIS2_PLACEMENT_3D ( 'NONE', #55510, #20221, #14599 ) ;
#29875=EDGE_CURVE ( 'NONE', #35686, #66579, #34480, .T. ) ;
#29893=DIRECTION ( 'NONE',  ( 0.000000000000000000, 0.000000000000000000, 1.000000000000000000 ) ) ;
#30085=VECTOR ( 'NONE', #35338, 1000.000000000000227 ) ;
#30249=EDGE_CURVE ( 'NONE', #12453, #66690, #67119, .T. ) ;
#30587=VERTEX_POINT ( 'NONE', #34108 ) ;
#30615=CIRCLE ( 'NONE', #27227, 200.0000000000000000 ) ;
#30617=EDGE_LOOP ( 'NONE', ( #51747, #54988, #33780, #63979, #32163, #42594 ) ) ;
#30702=AXIS2_PLACEMENT_3D ( 'NONE', #64951, #11460, #27297 ) ;
#30817=VECTOR ( 'NONE', #539, 1000.000000000000000 ) ;
#30908=DIRECTION ( 'NONE',  ( 1.000000000000000000, 0.000000000000000000, 0.000000000000000000 ) ) ;
#30925=CARTESIAN_POINT ( 'NONE',  ( -6.000000000000000000, 23.07878402833891229, -5.000000000000000000 ) ) ;
#30968=VECTOR ( 'NONE', #51368, 1000.000000000000000 ) ;
#31042=ADVANCED_FACE ( 'NONE', ( #8335 ), #23816, .F. ) ;
#31121=ORIENTED_EDGE ( 'NONE', *, *, #50441, .T. ) ;
#31221=FACE_BOUND ( 'NONE', #33575, .T. ) ;
#31328=DIRECTION ( 'NONE',  ( 1.000000000000000000, 0.000000000000000000, 0.000000000000000000 ) ) ;
#31513=LINE ( 'NONE', #48344, #32489 ) ;
#31698=EDGE_CURVE ( 'NONE', #14003, #64820, #50376, .T. ) ;
#31844=ADVANCED_FACE ( 'NONE', ( #18626 ), #40083, .F. ) ;
#32071=DIRECTION ( 'NONE',  ( -1.000000000000000000, 0.000000000000000000, 0.000000000000000000 ) ) ;
#32163=ORIENTED_EDGE ( 'NONE', *, *, #49764, .F. ) ;
#32190=DIRECTION ( 'NONE',  ( 0.000000000000000000, -0.000000000000000000, 1.000000000000000000 ) ) ;
#32255=LINE ( 'NONE', #27653, #26576 ) ;
#32271=EDGE_LOOP ( 'NONE', ( #49506, #2092, #20210, #39875 ) ) ;
#32328=ORIENTED_EDGE ( 'NONE', *, *, #64810, .F. ) ;
#32489=VECTOR ( 'NONE', #53290, 1000.000000000000000 ) ;
#32810=ORIENTED_EDGE ( 'NONE', *, *, #38176, .T. ) ;
#32890=DIRECTION ( 'NONE',  ( -0.000000000000000000, -0.000000000000000000, 1.000000000000000000 ) ) ;
#32902=AXIS2_PLACEMENT_3D ( 'NONE', #41423, #57600, #36488 ) ;
#32968=VECTOR ( 'NONE', #58131, 1000.000000000000000 ) ;
#33040=CARTESIAN_POINT ( 'NONE',  ( 0.000000000000000000, 65.13282190615278466, -9.999999999999998224 ) ) ;
#33075=CARTESIAN_POINT ( 'NONE',  ( 6.000000000000000000, 19.07878402833891229, -5.000000000000000888 ) ) ;
#33268=ADVANCED_BREP_SHAPE_REPRESENTATION ( '', ( #17922, #66832 ), #59007 ) ;
#33520=EDGE_LOOP ( 'NONE', ( #48650, #60012, #41861, #25296 ) ) ;
#33526=AXIS2_PLACEMENT_3D ( 'NONE', #47898, #27839, #10963 ) ;
#33572=CARTESIAN_POINT ( 'NONE',  ( 0.000000000000000000, 0.000000000000000000, 5.000000000000000000 ) ) ;
#33575=EDGE_LOOP ( 'NONE', ( #16044, #57389 ) ) ;
#33600=ORIENTED_EDGE ( 'NONE', *, *, #62973, .F. ) ;
#33780=ORIENTED_EDGE ( 'NONE', *, *, #27751, .F. ) ;
#33848=CARTESIAN_POINT ( 'NONE',  ( 20.00000000000000000, 0.000000000000000000, -5.000000000000000888 ) ) ;
#33867=ORIENTED_EDGE ( 'NONE', *, *, #48903, .T. ) ;
#33980=ADVANCED_FACE ( 'NONE', ( #53137 ), #64754, .F. ) ;
#34066=VECTOR ( 'NONE', #65480, 1000.000000000000000 ) ;
#34108=CARTESIAN_POINT ( 'NONE',  ( -125.0000000000000000, 0.000000000000000000, -10.00000000000000000 ) ) ;
#34186=VERTEX_POINT ( 'NONE', #42522 ) ;
#34341=VERTEX_POINT ( 'NONE', #17159 ) ;
#34464=ORIENTED_EDGE ( 'NONE', *, *, #18905, .F. ) ;
#34476=DIRECTION ( 'NONE',  ( 0.000000000000000000, 0.000000000000000000, 1.000000000000000000 ) ) ;
#34480=CIRCLE ( 'NONE', #15371, 185.0000000000000000 ) ;
#34498=CARTESIAN_POINT ( 'NONE',  ( 0.000000000000000000, 0.000000000000000000, 10.00000000000000000 ) ) ;
#34567=AXIS2_PLACEMENT_3D ( 'NONE', #8506, #39466, #66567 ) ;
#34629=CARTESIAN_POINT ( 'NONE',  ( -5.999999999999998224, 19.07878402833891229, -5.000000000000000000 ) ) ;
#34775=VERTEX_POINT ( 'NONE', #16915 ) ;
#34925=ORIENTED_EDGE ( 'NONE', *, *, #14558, .T. ) ;
#35077=ADVANCED_FACE ( 'NONE', ( #8817 ), #56645, .F. ) ;
#35090=EDGE_CURVE ( 'NONE', #66690, #47682, #14436, .T. ) ;
#35127=CARTESIAN_POINT ( 'NONE',  ( 185.0000000000000000, 0.000000000000000000, 0.000000000000000000 ) ) ;
#35149=CARTESIAN_POINT ( 'NONE',  ( 6.000000000000000000, 23.07878402833891229, -5.000000000000000000 ) ) ;
#35190=DIRECTION ( 'NONE',  ( -0.000000000000000000, 0.000000000000000000, -1.000000000000000000 ) ) ;
#35338=DIRECTION ( 'NONE',  ( -0.9578262852211514300, 0.000000000000000000, -0.2873478855663451625 ) ) ;
#35359=DIRECTION ( 'NONE',  ( -0.000000000000000000, -0.000000000000000000, 1.000000000000000000 ) ) ;
#35413=ADVANCED_FACE ( 'NONE', ( #51971 ), #25255, .F. ) ;
#35423=AXIS2_PLACEMENT_3D ( 'NONE', #62572, #58647, #30908 ) ;
#35502=LINE ( 'NONE', #35149, #800 ) ;
#35516=DIRECTION ( 'NONE',  ( -0.000000000000000000, -0.000000000000000000, 1.000000000000000000 ) ) ;
#35591=ORIENTED_EDGE ( 'NONE', *, *, #2182, .T. ) ;
#35686=VERTEX_POINT ( 'NONE', #23781 ) ;
#35863=EDGE_LOOP ( 'NONE', ( #14176, #44490, #65810, #22006 ) ) ;
#35886=CARTESIAN_POINT ( 'NONE',  ( -25.00000000000028066, -65.13282190615278466, -9.999999999999998224 ) ) ;
#35988=ORIENTED_EDGE ( 'NONE', *, *, #50811, .T. ) ;
#36085=ORIENTED_EDGE ( 'NONE', *, *, #13260, .T. ) ;
#36117=ORIENTED_EDGE ( 'NONE', *, *, #7935, .F. ) ;
#36135=LINE ( 'NONE', #57594, #57193 ) ;
#36195=LINE ( 'NONE', #30925, #30817 ) ;
#36222=EDGE_LOOP ( 'NONE', ( #43180, #59135, #59263, #44775 ) ) ;
#36232=DIRECTION ( 'NONE',  ( 1.000000000000000000, 0.000000000000000000, -0.000000000000000000 ) ) ;
#36325=CYLINDRICAL_SURFACE ( 'NONE', #53672, 185.0000000000000000 ) ;
#36379=VECTOR ( 'NONE', #52662, 1000.000000000000000 ) ;
#36386=EDGE_CURVE ( 'NONE', #383, #34775, #45243, .T. ) ;
#36428=CARTESIAN_POINT ( 'NONE',  ( 3.678442866637813759E-12, -65.13282190615278466, -9.999999999999998224 ) ) ;
#36434=ADVANCED_FACE ( 'NONE', ( #61762 ), #51574, .T. ) ;
#36458=DIRECTION ( 'NONE',  ( 1.000000000000000000, 0.000000000000000000, 0.000000000000000000 ) ) ;
#36481=CARTESIAN_POINT ( 'NONE',  ( 25.00000000000000000, 65.13282190615278466, -9.999999999999998224 ) ) ;
#36488=DIRECTION ( 'NONE',  ( 1.000000000000000000, 0.000000000000000000, -0.000000000000000000 ) ) ;
#36527=EDGE_LOOP ( 'NONE', ( #33600, #55070 ) ) ;
#36656=DIRECTION ( 'NONE',  ( 0.000000000000000000, 0.000000000000000000, 1.000000000000000000 ) ) ;
#36731=CIRCLE ( 'NONE', #23281, 125.0000000000000000 ) ;
#36794=DIRECTION ( 'NONE',  ( -0.000000000000000000, -0.000000000000000000, -1.000000000000000000 ) ) ;
#36849=CARTESIAN_POINT ( 'NONE',  ( 3.678442866637813759E-12, -65.13282190615278466, 5.000000000000000000 ) ) ;
#36926=ORIENTED_EDGE ( 'NONE', *, *, #36386, .F. ) ;
#36968=DIRECTION ( 'NONE',  ( 0.000000000000000000, 0.000000000000000000, 1.000000000000000000 ) ) ;
#37196=CARTESIAN_POINT ( 'NONE',  ( -200.0000000000000000, 2.449293598294706434E-14, -10.00000000000000000 ) ) ;
#37197=FILL_AREA_STYLE_COLOUR ( '', #66486 ) ;
#37271=MECHANICAL_DESIGN_GEOMETRIC_PRESENTATION_REPRESENTATION('',(#52978),#12588);
#37333=DIRECTION ( 'NONE',  ( 0.000000000000000000, 0.000000000000000000, -1.000000000000000000 ) ) ;
#37446=FACE_OUTER_BOUND ( 'NONE', #1338, .T. ) ;
#37463=AXIS2_PLACEMENT_3D ( 'NONE', #67065, #3977, #57785 ) ;
#37584=DIRECTION ( 'NONE',  ( 1.000000000000000000, 0.000000000000000000, 0.000000000000000000 ) ) ;
#37736=ORIENTED_EDGE ( 'NONE', *, *, #64384, .F. ) ;
#37879=CARTESIAN_POINT ( 'NONE',  ( 20.00000000000000000, 0.000000000000000000, 5.000000000000000000 ) ) ;
#38000=DIRECTION ( 'NONE',  ( 0.000000000000000000, 0.000000000000000000, 1.000000000000000000 ) ) ;
#38056=LINE ( 'NONE', #4663, #16034 ) ;
#38176=EDGE_CURVE ( 'NONE', #64281, #34186, #29443, .T. ) ;
#38209=AXIS2_PLACEMENT_3D ( 'NONE', #16296, #4368, #26852 ) ;
#38340=CARTESIAN_POINT ( 'NONE',  ( 0.000000000000000000, 0.000000000000000000, 2.499999999999999556 ) ) ;
#38346=DIRECTION ( 'NONE',  ( 1.000000000000000000, 0.000000000000000000, 0.000000000000000000 ) ) ;
#38355=DIRECTION ( 'NONE',  ( 0.000000000000000000, 0.000000000000000000, 1.000000000000000000 ) ) ;
#38568=CARTESIAN_POINT ( 'NONE',  ( 0.000000000000000000, 0.000000000000000000, 10.00000000000000000 ) ) ;
#38602=DIRECTION ( 'NONE',  ( -1.000000000000000000, 0.000000000000000000, 0.000000000000000000 ) ) ;
#38628=DIRECTION ( 'NONE',  ( -1.000000000000000000, 0.000000000000000000, 0.000000000000000000 ) ) ;
#38698=FACE_OUTER_BOUND ( 'NONE', #68739, .T. ) ;
#38961=CARTESIAN_POINT ( 'NONE',  ( 125.0000000000000000, 1.530808498934191561E-14, -10.00000000000000000 ) ) ;
#38969=DIRECTION ( 'NONE',  ( 0.000000000000000000, 0.000000000000000000, -1.000000000000000000 ) ) ;
#38989=CARTESIAN_POINT ( 'NONE',  ( 65.13282190615461786, 1.839221433318906476E-12, -5.000000000000000000 ) ) ;
#39156=DIRECTION ( 'NONE',  ( -0.000000000000000000, -0.000000000000000000, 1.000000000000000000 ) ) ;
#39203=VERTEX_POINT ( 'NONE', #44165 ) ;
#39236=CONICAL_SURFACE ( 'NONE', #66219, 200.0000000000000000, 1.279339532317029793 ) ;
#39239=ADVANCED_FACE ( 'NONE', ( #10776 ), #53681, .F. ) ;
#39305=DIRECTION ( 'NONE',  ( 0.000000000000000000, 0.000000000000000000, -1.000000000000000000 ) ) ;
#39365=EDGE_LOOP ( 'NONE', ( #53221, #59036, #34925, #6627 ) ) ;
#39383=CARTESIAN_POINT ( 'NONE',  ( -200.0000000000000000, 2.449293598294706434E-14, -10.00000000000000000 ) ) ;
#39406=CARTESIAN_POINT ( 'NONE',  ( 0.000000000000000000, 0.000000000000000000, -10.00000000000000000 ) ) ;
#39466=DIRECTION ( 'NONE',  ( 0.000000000000000000, 0.000000000000000000, 1.000000000000000000 ) ) ;
#39478=ORIENTED_EDGE ( 'NONE', *, *, #47800, .T. ) ;
#39536=CARTESIAN_POINT ( 'NONE',  ( 25.00000000000763478, -65.13282190615278466, -5.000000000000000000 ) ) ;
#39557=EDGE_CURVE ( 'NONE', #64281, #23906, #54554, .T. ) ;
#39560=AXIS2_PLACEMENT_3D ( 'NONE', #359, #38000, #38346 ) ;
#39728=LINE ( 'NONE', #18273, #26713 ) ;
#39742=CIRCLE ( 'NONE', #13927, 25.00000000000000000 ) ;
#39875=ORIENTED_EDGE ( 'NONE', *, *, #49221, .T. ) ;
#39938=DIRECTION ( 'NONE',  ( 1.000000000000000000, 0.000000000000000000, 0.000000000000000000 ) ) ;
#40083=CYLINDRICAL_SURFACE ( 'NONE', #59344, 25.00000000000395772 ) ;
#40146=ORIENTED_EDGE ( 'NONE', *, *, #64810, .T. ) ;
#40193=DIRECTION ( 'NONE',  ( 0.000000000000000000, 0.000000000000000000, 1.000000000000000000 ) ) ;
#40229=AXIS2_PLACEMENT_3D ( 'NONE', #45428, #12731, #29257 ) ;
#40260=VERTEX_POINT ( 'NONE', #37879 ) ;
#40316=DIRECTION ( 'NONE',  ( 0.9578262852211514300, 1.172998894335282758E-16, -0.2873478855663451625 ) ) ;
#40323=CARTESIAN_POINT ( 'NONE',  ( 0.000000000000000000, 65.13282190615278466, 5.000000000000000000 ) ) ;
#40349=DIRECTION ( 'NONE',  ( 1.000000000000000000, 0.000000000000000000, 0.000000000000000000 ) ) ;
#40367=CARTESIAN_POINT ( 'NONE',  ( -20.00000000000000000, 2.449293598294706513E-15, -5.000000000000000888 ) ) ;
#40401=LINE ( 'NONE', #35127, #15085 ) ;
#40484=CARTESIAN_POINT ( 'NONE',  ( 0.000000000000000000, 0.000000000000000000, -5.000000000000000000 ) ) ;
#40661=DIRECTION ( 'NONE',  ( 0.000000000000000000, 0.000000000000000000, 1.000000000000000000 ) ) ;
#40801=CARTESIAN_POINT ( 'NONE',  ( 6.000000000000000000, 19.07878402833891229, -20.00000000000000000 ) ) ;
#41143=AXIS2_PLACEMENT_3D ( 'NONE', #38340, #59783, #11594 ) ;
#41177=CARTESIAN_POINT ( 'NONE',  ( 40.13282190615316836, 1.842283050316774879E-12, -5.000000000000000000 ) ) ;
#41216=ADVANCED_FACE ( 'NONE', ( #46280, #3047 ), #19201, .T. ) ;
#41423=CARTESIAN_POINT ( 'NONE',  ( 0.000000000000000000, 0.000000000000000000, 5.000000000000000000 ) ) ;
#41456=( NAMED_UNIT ( * ) PLANE_ANGLE_UNIT ( ) SI_UNIT ( $, .RADIAN. ) );
#41500=VERTEX_POINT ( 'NONE', #46900 ) ;
#41666=EDGE_LOOP ( 'NONE', ( #47859, #64047 ) ) ;
#41706=CYLINDRICAL_SURFACE ( 'NONE', #12948, 25.00000000000395772 ) ;
#41765=FACE_BOUND ( 'NONE', #54432, .T. ) ;
#41790=ORIENTED_EDGE ( 'NONE', *, *, #2182, .F. ) ;
#41861=ORIENTED_EDGE ( 'NONE', *, *, #23699, .T. ) ;
#41922=DIRECTION ( 'NONE',  ( -0.000000000000000000, -0.000000000000000000, 1.000000000000000000 ) ) ;
#41925=CARTESIAN_POINT ( 'NONE',  ( 0.000000000000000000, 0.000000000000000000, -10.00000000000000000 ) ) ;
#42056=DIRECTION ( 'NONE',  ( 1.000000000000000000, 0.000000000000000000, 0.000000000000000000 ) ) ;
#42062=FACE_OUTER_BOUND ( 'NONE', #61016, .T. ) ;
#42097=AXIS2_PLACEMENT_3D ( 'NONE', #51187, #9656, #29723 ) ;
#42100=ORIENTED_EDGE ( 'NONE', *, *, #7432, .T. ) ;
#42291=DIRECTION ( 'NONE',  ( -0.000000000000000000, -0.000000000000000000, 1.000000000000000000 ) ) ;
#42294=AXIS2_PLACEMENT_3D ( 'NONE', #45958, #36794, #19217 ) ;
#42362=DIRECTION ( 'NONE',  ( 0.000000000000000000, 0.000000000000000000, 1.000000000000000000 ) ) ;
#42409=DIRECTION ( 'NONE',  ( 0.000000000000000000, 0.000000000000000000, 1.000000000000000000 ) ) ;
#42414=EDGE_LOOP ( 'NONE', ( #20277, #14562, #52682, #46406 ) ) ;
#42522=CARTESIAN_POINT ( 'NONE',  ( -90.13282190615392153, -1.844136286507718230E-12, -5.000000000000000000 ) ) ;
#42594=ORIENTED_EDGE ( 'NONE', *, *, #55396, .F. ) ;
#42657=ORIENTED_EDGE ( 'NONE', *, *, #14558, .F. ) ;
#42660=CARTESIAN_POINT ( 'NONE',  ( -185.0000000000000000, 2.265596578422603396E-14, -2.500000000000002220 ) ) ;
#42690=AXIS2_PLACEMENT_3D ( 'NONE', #62264, #36232, #35190 ) ;
#42884=EDGE_LOOP ( 'NONE', ( #36085, #44147, #19149, #41790 ) ) ;
#42994=ORIENTED_EDGE ( 'NONE', *, *, #18905, .T. ) ;
#43059=ORIENTED_EDGE ( 'NONE', *, *, #2575, .T. ) ;
#43062=( NAMED_UNIT ( * ) PLANE_ANGLE_UNIT ( ) SI_UNIT ( $, .RADIAN. ) );
#43180=ORIENTED_EDGE ( 'NONE', *, *, #47563, .F. ) ;
#43198=EDGE_LOOP ( 'NONE', ( #5861, #65959, #67196, #65125 ) ) ;
#43482=EDGE_CURVE ( 'NONE', #13178, #64820, #14594, .T. ) ;
#43509=LINE ( 'NONE', #53716, #59904 ) ;
#43541=ORIENTED_EDGE ( 'NONE', *, *, #31698, .F. ) ;
#43794=CARTESIAN_POINT ( 'NONE',  ( -5.999999999999998224, 19.07878402833891229, 4.999999999999997335 ) ) ;
#43795=DIRECTION ( 'NONE',  ( 1.000000000000000000, 0.000000000000000000, 0.000000000000000000 ) ) ;
#44147=ORIENTED_EDGE ( 'NONE', *, *, #67936, .F. ) ;
#44165=CARTESIAN_POINT ( 'NONE',  ( -90.13282190615392153, -1.844136286507718230E-12, 5.000000000000000000 ) ) ;
#44365=ORIENTED_EDGE ( 'NONE', *, *, #60097, .F. ) ;
#44391=AXIS2_PLACEMENT_3D ( 'NONE', #68647, #41922, #52132 ) ;
#44397=CIRCLE ( 'NONE', #619, 200.0000000000000000 ) ;
#44434=CARTESIAN_POINT ( 'NONE',  ( 90.13282190615606737, 1.839221433318906476E-12, -9.999999999999998224 ) ) ;
#44490=ORIENTED_EDGE ( 'NONE', *, *, #61188, .T. ) ;
#44492=ORIENTED_EDGE ( 'NONE', *, *, #68141, .T. ) ;
#44558=DIRECTION ( 'NONE',  ( 0.000000000000000000, 0.000000000000000000, 1.000000000000000000 ) ) ;
#44620=DIRECTION ( 'NONE',  ( 1.000000000000000000, 0.000000000000000000, 0.000000000000000000 ) ) ;
#44634=EDGE_CURVE ( 'NONE', #29280, #22360, #16367, .T. ) ;
#44670=DIRECTION ( 'NONE',  ( 1.000000000000000000, 0.000000000000000000, 0.000000000000000000 ) ) ;
#44673=DIRECTION ( 'NONE',  ( -1.000000000000000000, 0.000000000000000000, 0.000000000000000000 ) ) ;
#44716=ORIENTED_EDGE ( 'NONE', *, *, #2575, .F. ) ;
#44725=ADVANCED_FACE ( 'NONE', ( #28335 ), #7933, .F. ) ;
#44738=ORIENTED_EDGE ( 'NONE', *, *, #7935, .T. ) ;
#44759=ORIENTED_EDGE ( 'NONE', *, *, #39557, .T. ) ;
#44775=ORIENTED_EDGE ( 'NONE', *, *, #58138, .F. ) ;
#45000=CARTESIAN_POINT ( 'NONE',  ( 0.000000000000000000, 0.000000000000000000, 10.00000000000000000 ) ) ;
#45079=EDGE_CURVE ( 'NONE', #56426, #1003, #67012, .T. ) ;
#45221=ORIENTED_EDGE ( 'NONE', *, *, #7432, .F. ) ;
#45243=LINE ( 'NONE', #7631, #50634 ) ;
#45372=CIRCLE ( 'NONE', #63351, 25.00000000000145306 ) ;
#45428=CARTESIAN_POINT ( 'NONE',  ( 0.000000000000000000, 0.000000000000000000, -7.000000000000000000 ) ) ;
#45507=AXIS2_PLACEMENT_3D ( 'NONE', #50067, #65202, #11727 ) ;
#45550=AXIS2_PLACEMENT_3D ( 'NONE', #2164, #8477, #67917 ) ;
#45668=EDGE_CURVE ( 'NONE', #19424, #27213, #10174, .T. ) ;
#45707=DIRECTION ( 'NONE',  ( 1.000000000000000000, 0.000000000000000000, 0.000000000000000000 ) ) ;
#45849=EDGE_LOOP ( 'NONE', ( #28061, #7395, #19225, #9932 ) ) ;
#45858=ORIENTED_EDGE ( 'NONE', *, *, #66289, .F. ) ;
#45958=CARTESIAN_POINT ( 'NONE',  ( 0.000000000000000000, 0.000000000000000000, -5.000000000000000000 ) ) ;
#46028=DIRECTION ( 'NONE',  ( -0.000000000000000000, -0.000000000000000000, -1.000000000000000000 ) ) ;
#46211=CIRCLE ( 'NONE', #20402, 20.00000000000000000 ) ;
#46240=ORIENTED_EDGE ( 'NONE', *, *, #48903, .F. ) ;
#46280=FACE_BOUND ( 'NONE', #7683, .T. ) ;
#46311=CARTESIAN_POINT ( 'NONE',  ( -65.13282190615095146, -1.847197903505587038E-12, 5.000000000000000000 ) ) ;
#46406=ORIENTED_EDGE ( 'NONE', *, *, #43482, .F. ) ;
#46584=VERTEX_POINT ( 'NONE', #23277 ) ;
#46638=ORIENTED_EDGE ( 'NONE', *, *, #56377, .F. ) ;
#46640=PRODUCT_CONTEXT ( 'NONE', #48895, 'mechanical' ) ;
#46681=FACE_BOUND ( 'NONE', #15924, .T. ) ;
#46688=FACE_BOUND ( 'NONE', #68032, .T. ) ;
#46691=DIRECTION ( 'NONE',  ( -0.000000000000000000, -0.000000000000000000, 1.000000000000000000 ) ) ;
#46702=DIRECTION ( 'NONE',  ( 0.000000000000000000, 0.000000000000000000, 1.000000000000000000 ) ) ;
#46900=CARTESIAN_POINT ( 'NONE',  ( -125.0000000000000000, 0.000000000000000000, -5.000000000000000000 ) ) ;
#47238=EDGE_LOOP ( 'NONE', ( #27043, #9736, #44738, #7148 ) ) ;
#47331=EDGE_LOOP ( 'NONE', ( #14006, #26076 ) ) ;
#47366=FACE_BOUND ( 'NONE', #36527, .T. ) ;
#47416=ORIENTED_EDGE ( 'NONE', *, *, #58138, .T. ) ;
#47563=EDGE_CURVE ( 'NONE', #35686, #61651, #53443, .T. ) ;
#47605=AXIS2_PLACEMENT_3D ( 'NONE', #65346, #38969, #5890 ) ;
#47656=PLANE ( 'NONE',  #19655 ) ;
#47682=VERTEX_POINT ( 'NONE', #58722 ) ;
#47800=EDGE_CURVE ( 'NONE', #34186, #64281, #4276, .T. ) ;
#47848=DIRECTION ( 'NONE',  ( -1.000000000000000000, 0.000000000000000000, 0.000000000000000000 ) ) ;
#47859=ORIENTED_EDGE ( 'NONE', *, *, #66822, .T. ) ;
#47898=CARTESIAN_POINT ( 'NONE',  ( 0.000000000000000000, 0.000000000000000000, -10.00000000000000000 ) ) ;
#47923=CARTESIAN_POINT ( 'NONE',  ( 0.000000000000000000, 23.07878402833891229, 5.000000000000000000 ) ) ;
#47964=CYLINDRICAL_SURFACE ( 'NONE', #15442, 20.00000000000000000 ) ;
#48117=EDGE_LOOP ( 'NONE', ( #24969, #42994 ) ) ;
#48120=ADVANCED_FACE ( 'NONE', ( #56329 ), #16610, .T. ) ;
#48133=ORIENTED_EDGE ( 'NONE', *, *, #58327, .F. ) ;
#48183=CARTESIAN_POINT ( 'NONE',  ( -6.000000000000000000, 23.07878402833891229, 9.999999999999998224 ) ) ;
#48344=CARTESIAN_POINT ( 'NONE',  ( 25.00000000000763478, -65.13282190615278466, -9.999999999999998224 ) ) ;
#48378=DIRECTION ( 'NONE',  ( -0.000000000000000000, 1.000000000000000000, -0.000000000000000000 ) ) ;
#48447=ORIENTED_EDGE ( 'NONE', *, *, #52622, .F. ) ;
#48453=EDGE_CURVE ( 'NONE', #54841, #35686, #39728, .T. ) ;
#48533=CYLINDRICAL_SURFACE ( 'NONE', #203, 200.0000000000000000 ) ;
#48586=CARTESIAN_POINT ( 'NONE',  ( 3.678442866637813759E-12, -65.13282190615278466, -5.000000000000000000 ) ) ;
#48650=ORIENTED_EDGE ( 'NONE', *, *, #48453, .F. ) ;
#48814=VERTEX_POINT ( 'NONE', #66404 ) ;
#48842=VERTEX_POINT ( 'NONE', #38961 ) ;
#48865=VERTEX_POINT ( 'NONE', #28388 ) ;
#48879=CIRCLE ( 'NONE', #45550, 20.00000000000000000 ) ;
#48895=APPLICATION_CONTEXT ( 'automotive_design' ) ;
#48902=EDGE_CURVE ( 'NONE', #27213, #46584, #63433, .T. ) ;
#48903=EDGE_CURVE ( 'NONE', #34186, #39203, #25808, .T. ) ;
#48948=AXIS2_PLACEMENT_3D ( 'NONE', #15539, #58429, #53140 ) ;
#49077=DIRECTION ( 'NONE',  ( 1.000000000000000000, 0.000000000000000000, 0.000000000000000000 ) ) ;
#49132=CARTESIAN_POINT ( 'NONE',  ( 0.000000000000000000, 0.000000000000000000, -7.000000000000000000 ) ) ;
#49206=CIRCLE ( 'NONE', #33526, 125.0000000000000000 ) ;
#49221=EDGE_CURVE ( 'NONE', #50826, #22538, #16554, .T. ) ;
#49232=VERTEX_POINT ( 'NONE', #33848 ) ;
#49270=EDGE_LOOP ( 'NONE', ( #63317, #26151 ) ) ;
#49506=ORIENTED_EDGE ( 'NONE', *, *, #21663, .F. ) ;
#49567=LINE ( 'NONE', #39383, #56053 ) ;
#49581=VERTEX_POINT ( 'NONE', #711 ) ;
#49601=ORIENTED_EDGE ( 'NONE', *, *, #45079, .T. ) ;
#49689=ORIENTED_EDGE ( 'NONE', *, *, #13273, .T. ) ;
#49723=VECTOR ( 'NONE', #48378, 1000.000000000000000 ) ;
#49764=EDGE_CURVE ( 'NONE', #23613, #25857, #35502, .T. ) ;
#49810=CARTESIAN_POINT ( 'NONE',  ( 200.0000000000000000, 0.000000000000000000, -10.00000000000000000 ) ) ;
#49816=CIRCLE ( 'NONE', #19500, 25.00000000000395772 ) ;
#49898=CARTESIAN_POINT ( 'NONE',  ( 0.000000000000000000, 0.000000000000000000, -5.000000000000000000 ) ) ;
#49925=AXIS2_PLACEMENT_3D ( 'NONE', #46311, #50908, #36458 ) ;
#50045=CYLINDRICAL_SURFACE ( 'NONE', #18205, 20.00000000000000000 ) ;
#50067=CARTESIAN_POINT ( 'NONE',  ( 0.000000000000000000, 65.13282190615278466, -9.999999999999998224 ) ) ;
#50169=VECTOR ( 'NONE', #21760, 1000.000000000000000 ) ;
#50247=CARTESIAN_POINT ( 'NONE',  ( 0.000000000000000000, 0.000000000000000000, -7.000000000000000000 ) ) ;
#50292=AXIS2_PLACEMENT_3D ( 'NONE', #41925, #36656, #3954 ) ;
#50376=CIRCLE ( 'NONE', #29045, 200.0000000000000000 ) ;
#50398=FACE_OUTER_BOUND ( 'NONE', #39365, .T. ) ;
#50401=CARTESIAN_POINT ( 'NONE',  ( 65.13282190615461786, 1.839221433318906476E-12, 5.000000000000000000 ) ) ;
#50441=EDGE_CURVE ( 'NONE', #54841, #16199, #51172, .T. ) ;
#50530=CARTESIAN_POINT ( 'NONE',  ( 0.000000000000000000, 0.000000000000000000, 0.000000000000000000 ) ) ;
#50621=ORIENTED_EDGE ( 'NONE', *, *, #22251, .F. ) ;
#50634=VECTOR ( 'NONE', #40316, 1000.000000000000227 ) ;
#50690=AXIS2_PLACEMENT_3D ( 'NONE', #26153, #69042, #10305 ) ;
#50717=CARTESIAN_POINT ( 'NONE',  ( -200.0000000000000000, 2.449293598294706434E-14, 7.000000000000000000 ) ) ;
#50728=ORIENTED_EDGE ( 'NONE', *, *, #14, .T. ) ;
#50796=AXIS2_PLACEMENT_3D ( 'NONE', #34498, #29893, #3504 ) ;
#50811=EDGE_CURVE ( 'NONE', #22360, #29280, #19209, .T. ) ;
#50826=VERTEX_POINT ( 'NONE', #43794 ) ;
#50838=CARTESIAN_POINT ( 'NONE',  ( 0.000000000000000000, 0.000000000000000000, -10.00000000000000000 ) ) ;
#50908=DIRECTION ( 'NONE',  ( 0.000000000000000000, 0.000000000000000000, 1.000000000000000000 ) ) ;
#50938=DIRECTION ( 'NONE',  ( 1.000000000000000000, 0.000000000000000000, 0.000000000000000000 ) ) ;
#51049=FACE_OUTER_BOUND ( 'NONE', #11237, .T. ) ;
#51098=AXIS2_PLACEMENT_3D ( 'NONE', #57200, #51579, #51231 ) ;
#51172=LINE ( 'NONE', #51520, #30085 ) ;
#51187=CARTESIAN_POINT ( 'NONE',  ( 0.000000000000000000, 0.000000000000000000, -5.000000000000000000 ) ) ;
#51231=DIRECTION ( 'NONE',  ( 1.000000000000000000, 0.000000000000000000, 0.000000000000000000 ) ) ;
#51368=DIRECTION ( 'NONE',  ( 0.000000000000000000, 0.000000000000000000, -1.000000000000000000 ) ) ;
#51520=CARTESIAN_POINT ( 'NONE',  ( -200.0000000000000000, 0.000000000000000000, -7.000000000000000000 ) ) ;
#51557=CARTESIAN_POINT ( 'NONE',  ( -20.00000000000000000, 2.449293598294706513E-15, -20.00000000000000000 ) ) ;
#51574=CYLINDRICAL_SURFACE ( 'NONE', #68608, 185.0000000000000000 ) ;
#51579=DIRECTION ( 'NONE',  ( 0.000000000000000000, 0.000000000000000000, 1.000000000000000000 ) ) ;
#51616=VECTOR ( 'NONE', #52645, 1000.000000000000000 ) ;
#51623=DIRECTION ( 'NONE',  ( 0.000000000000000000, 0.000000000000000000, 1.000000000000000000 ) ) ;
#51665=SURFACE_STYLE_FILL_AREA ( #8766 ) ;
#51747=ORIENTED_EDGE ( 'NONE', *, *, #856, .F. ) ;
#51971=FACE_OUTER_BOUND ( 'NONE', #23529, .T. ) ;
#52001=( LENGTH_UNIT ( ) NAMED_UNIT ( * ) SI_UNIT ( .MILLI., .METRE. ) );
#52132=DIRECTION ( 'NONE',  ( 1.000000000000000000, 0.000000000000000000, 0.000000000000000000 ) ) ;
#52136=CYLINDRICAL_SURFACE ( 'NONE', #50292, 200.0000000000000000 ) ;
#52341=PRODUCT_DEFINITION_FORMATION_WITH_SPECIFIED_SOURCE ( 'ANY', '', #6321, .NOT_KNOWN. ) ;
#52424=DIRECTION ( 'NONE',  ( 0.000000000000000000, 0.000000000000000000, -1.000000000000000000 ) ) ;
#52497=EDGE_CURVE ( 'NONE', #16199, #34775, #30615, .T. ) ;
#52614=VECTOR ( 'NONE', #63783, 1000.000000000000000 ) ;
#52622=EDGE_CURVE ( 'NONE', #66690, #12453, #2543, .T. ) ;
#52645=DIRECTION ( 'NONE',  ( -0.000000000000000000, -0.000000000000000000, 1.000000000000000000 ) ) ;
#52662=DIRECTION ( 'NONE',  ( 0.000000000000000000, 0.000000000000000000, 1.000000000000000000 ) ) ;
#52682=ORIENTED_EDGE ( 'NONE', *, *, #66822, .F. ) ;
#52978=STYLED_ITEM ( 'NONE', ( #19645 ), #17922 ) ;
#53001=DIRECTION ( 'NONE',  ( 0.000000000000000000, 0.000000000000000000, 1.000000000000000000 ) ) ;
#53079=CIRCLE ( 'NONE', #4792, 185.0000000000000000 ) ;
#53137=FACE_OUTER_BOUND ( 'NONE', #35863, .T. ) ;
#53140=DIRECTION ( 'NONE',  ( 1.000000000000000000, 0.000000000000000000, 0.000000000000000000 ) ) ;
#53221=ORIENTED_EDGE ( 'NONE', *, *, #27751, .T. ) ;
#53224=CIRCLE ( 'NONE', #47605, 20.00000000000000000 ) ;
#53269=( LENGTH_UNIT ( ) NAMED_UNIT ( * ) SI_UNIT ( .MILLI., .METRE. ) );
#53290=DIRECTION ( 'NONE',  ( -0.000000000000000000, -0.000000000000000000, 1.000000000000000000 ) ) ;
#53443=LINE ( 'NONE', #5272, #9853 ) ;
#53672=AXIS2_PLACEMENT_3D ( 'NONE', #20831, #42291, #9594 ) ;
#53681=CYLINDRICAL_SURFACE ( 'NONE', #30702, 25.00000000000296296 ) ;
#53716=CARTESIAN_POINT ( 'NONE',  ( -25.00000000000000000, 65.13282190615278466, -9.999999999999998224 ) ) ;
#53925=DIRECTION ( 'NONE',  ( 0.000000000000000000, 0.000000000000000000, 1.000000000000000000 ) ) ;
#53934=CARTESIAN_POINT ( 'NONE',  ( 6.000000000000000000, 23.07878402833891229, 5.000000000000000000 ) ) ;
#53954=CARTESIAN_POINT ( 'NONE',  ( -6.000000000000000000, 23.07878402833891229, 9.999999999999998224 ) ) ;
#53971=ORIENTED_EDGE ( 'NONE', *, *, #35090, .F. ) ;
#54034=CARTESIAN_POINT ( 'NONE',  ( 125.0000000000000000, 0.000000000000000000, 10.00000000000000000 ) ) ;
#54101=EDGE_CURVE ( 'NONE', #15739, #56426, #43509, .T. ) ;
#54114=ORIENTED_EDGE ( 'NONE', *, *, #23699, .F. ) ;
#54117=DIRECTION ( 'NONE',  ( 1.000000000000000000, 0.000000000000000000, 0.000000000000000000 ) ) ;
#54120=ORIENTED_EDGE ( 'NONE', *, *, #68379, .F. ) ;
#54135=EDGE_LOOP ( 'NONE', ( #24429, #1238 ) ) ;
#54327=DIRECTION ( 'NONE',  ( 1.000000000000000000, 0.000000000000000000, 0.000000000000000000 ) ) ;
#54432=EDGE_LOOP ( 'NONE', ( #18163, #63492, #22135, #56830, #42657, #67159 ) ) ;
#54551=EDGE_LOOP ( 'NONE', ( #34464, #17736, #11388, #7185 ) ) ;
#54554=LINE ( 'NONE', #12358, #34066 ) ;
#54571=AXIS2_PLACEMENT_3D ( 'NONE', #65199, #53925, #59900 ) ;
#54831=DIRECTION ( 'NONE',  ( 1.000000000000000000, 0.000000000000000000, 0.000000000000000000 ) ) ;
#54841=VERTEX_POINT ( 'NONE', #42660 ) ;
#54921=CARTESIAN_POINT ( 'NONE',  ( 0.000000000000000000, 65.13282190615278466, -5.000000000000000000 ) ) ;
#54923=CIRCLE ( 'NONE', #38209, 185.0000000000000000 ) ;
#54964=DIRECTION ( 'NONE',  ( 1.000000000000000000, 0.000000000000000000, 0.000000000000000000 ) ) ;
#54988=ORIENTED_EDGE ( 'NONE', *, *, #5568, .F. ) ;
#55070=ORIENTED_EDGE ( 'NONE', *, *, #68976, .F. ) ;
#55108=ORIENTED_EDGE ( 'NONE', *, *, #3365, .F. ) ;
#55130=CARTESIAN_POINT ( 'NONE',  ( 185.0000000000000000, 0.000000000000000000, -2.500000000000002220 ) ) ;
#55151=ORIENTED_EDGE ( 'NONE', *, *, #54101, .F. ) ;
#55185=CARTESIAN_POINT ( 'NONE',  ( 6.000000000000000000, 23.07878402833891229, -5.000000000000000000 ) ) ;
#55225=CYLINDRICAL_SURFACE ( 'NONE', #19352, 200.0000000000000000 ) ;
#55396=EDGE_CURVE ( 'NONE', #55490, #23613, #36195, .T. ) ;
#55407=ORIENTED_EDGE ( 'NONE', *, *, #68976, .T. ) ;
#55413=CARTESIAN_POINT ( 'NONE',  ( 0.000000000000000000, 0.000000000000000000, 5.000000000000000000 ) ) ;
#55490=VERTEX_POINT ( 'NONE', #12848 ) ;
#55510=CARTESIAN_POINT ( 'NONE',  ( 65.13282190615461786, 1.839221433318906476E-12, -9.999999999999998224 ) ) ;
#55517=ORIENTED_EDGE ( 'NONE', *, *, #24805, .F. ) ;
#55553=DIRECTION ( 'NONE',  ( 0.000000000000000000, 0.000000000000000000, 1.000000000000000000 ) ) ;
#55554=CIRCLE ( 'NONE', #49925, 25.00000000000296296 ) ;
#55593=ORIENTED_EDGE ( 'NONE', *, *, #52497, .T. ) ;
#55761=CIRCLE ( 'NONE', #19817, 20.00000000000000000 ) ;
#55813=FACE_OUTER_BOUND ( 'NONE', #56384, .T. ) ;
#56046=ORIENTED_EDGE ( 'NONE', *, *, #45079, .F. ) ;
#56053=VECTOR ( 'NONE', #55553, 1000.000000000000000 ) ;
#56124=ORIENTED_EDGE ( 'NONE', *, *, #54101, .T. ) ;
#56252=DIRECTION ( 'NONE',  ( -0.000000000000000000, -0.000000000000000000, 1.000000000000000000 ) ) ;
#56316=FACE_BOUND ( 'NONE', #13063, .T. ) ;
#56329=FACE_OUTER_BOUND ( 'NONE', #1566, .T. ) ;
#56377=EDGE_CURVE ( 'NONE', #23906, #39203, #55554, .T. ) ;
#56384=EDGE_LOOP ( 'NONE', ( #25215, #9344, #5134, #42100 ) ) ;
#56426=VERTEX_POINT ( 'NONE', #69142 ) ;
#56554=AXIS2_PLACEMENT_3D ( 'NONE', #38568, #53001, #22391 ) ;
#56634=ORIENTED_EDGE ( 'NONE', *, *, #68141, .F. ) ;
#56645=PLANE ( 'NONE',  #42690 ) ;
#56830=ORIENTED_EDGE ( 'NONE', *, *, #19397, .F. ) ;
#56871=AXIS2_PLACEMENT_3D ( 'NONE', #48183, #47848, #36968 ) ;
#56912=FACE_OUTER_BOUND ( 'NONE', #48117, .T. ) ;
#57077=EDGE_CURVE ( 'NONE', #11859, #48814, #62239, .T. ) ;
#57193=VECTOR ( 'NONE', #68488, 1000.000000000000000 ) ;
#57200=CARTESIAN_POINT ( 'NONE',  ( 3.678442866637813759E-12, -65.13282190615278466, 5.000000000000000000 ) ) ;
#57238=AXIS2_PLACEMENT_3D ( 'NONE', #14671, #51623, #57245 ) ;
#57245=DIRECTION ( 'NONE',  ( 1.000000000000000000, 0.000000000000000000, -0.000000000000000000 ) ) ;
#57294=LINE ( 'NONE', #20009, #28792 ) ;
#57389=ORIENTED_EDGE ( 'NONE', *, *, #6603, .F. ) ;
#57497=DIRECTION ( 'NONE',  ( 0.000000000000000000, 0.000000000000000000, 1.000000000000000000 ) ) ;
#57510=CARTESIAN_POINT ( 'NONE',  ( 200.0000000000000000, 0.000000000000000000, -10.00000000000000000 ) ) ;
#57589=ORIENTED_EDGE ( 'NONE', *, *, #22064, .T. ) ;
#57594=CARTESIAN_POINT ( 'NONE',  ( -6.000000000000000000, 0.000000000000000000, 5.000000000000000000 ) ) ;
#57600=DIRECTION ( 'NONE',  ( 0.000000000000000000, 0.000000000000000000, 1.000000000000000000 ) ) ;
#57673=CYLINDRICAL_SURFACE ( 'NONE', #18759, 20.00000000000000000 ) ;
#57726=ORIENTED_EDGE ( 'NONE', *, *, #36386, .T. ) ;
#57785=DIRECTION ( 'NONE',  ( 1.000000000000000000, 0.000000000000000000, 0.000000000000000000 ) ) ;
#57861=LINE ( 'NONE', #51557, #7149 ) ;
#57883=DIRECTION ( 'NONE',  ( -0.000000000000000000, -0.000000000000000000, 1.000000000000000000 ) ) ;
#57938=PLANE ( 'NONE',  #32902 ) ;
#58045=ORIENTED_EDGE ( 'NONE', *, *, #11570, .T. ) ;
#58099=ORIENTED_EDGE ( 'NONE', *, *, #47563, .T. ) ;
#58131=DIRECTION ( 'NONE',  ( -0.000000000000000000, -0.000000000000000000, -1.000000000000000000 ) ) ;
#58138=EDGE_CURVE ( 'NONE', #61651, #13178, #17536, .T. ) ;
#58241=VECTOR ( 'NONE', #20508, 1000.000000000000000 ) ;
#58327=EDGE_CURVE ( 'NONE', #27213, #23613, #22194, .T. ) ;
#58375=ADVANCED_FACE ( 'NONE', ( #6362 ), #62494, .T. ) ;
#58429=DIRECTION ( 'NONE',  ( -0.000000000000000000, -0.000000000000000000, 1.000000000000000000 ) ) ;
#58441=CARTESIAN_POINT ( 'NONE',  ( 0.000000000000000000, 0.000000000000000000, -5.000000000000000888 ) ) ;
#58642=( NAMED_UNIT ( * ) SI_UNIT ( $, .STERADIAN. ) SOLID_ANGLE_UNIT ( ) );
#58647=DIRECTION ( 'NONE',  ( 0.000000000000000000, 0.000000000000000000, 1.000000000000000000 ) ) ;
#58722=CARTESIAN_POINT ( 'NONE',  ( -25.00000000000028066, -65.13282190615278466, 5.000000000000000000 ) ) ;
#58767=DIRECTION ( 'NONE',  ( -1.000000000000000000, 0.000000000000000000, 0.000000000000000000 ) ) ;
#58887=ADVANCED_FACE ( 'NONE', ( #23352 ), #7158, .F. ) ;
#59007=( GEOMETRIC_REPRESENTATION_CONTEXT ( 3 ) GLOBAL_UNCERTAINTY_ASSIGNED_CONTEXT ( ( #12116 ) ) GLOBAL_UNIT_ASSIGNED_CONTEXT ( ( #53269, #43062, #26898 ) ) REPRESENTATION_CONTEXT ( 'NONE', 'WORKASPACE' ) );
#59036=ORIENTED_EDGE ( 'NONE', *, *, #21663, .T. ) ;
#59128=EDGE_CURVE ( 'NONE', #25857, #49232, #55761, .T. ) ;
#59135=ORIENTED_EDGE ( 'NONE', *, *, #29875, .T. ) ;
#59150=ORIENTED_EDGE ( 'NONE', *, *, #3280, .F. ) ;
#59263=ORIENTED_EDGE ( 'NONE', *, *, #3280, .T. ) ;
#59286=CARTESIAN_POINT ( 'NONE',  ( 0.000000000000000000, 0.000000000000000000, -10.00000000000000000 ) ) ;
#59296=DIRECTION ( 'NONE',  ( 0.000000000000000000, 0.000000000000000000, 1.000000000000000000 ) ) ;
#59305=CARTESIAN_POINT ( 'NONE',  ( -6.000000000000000000, 23.07878402833891229, -5.000000000000000000 ) ) ;
#59344=AXIS2_PLACEMENT_3D ( 'NONE', #13357, #56252, #45707 ) ;
#59454=DIRECTION ( 'NONE',  ( 1.000000000000000000, 0.000000000000000000, 0.000000000000000000 ) ) ;
#59624=DIRECTION ( 'NONE',  ( 0.000000000000000000, 0.000000000000000000, 1.000000000000000000 ) ) ;
#59651=DIRECTION ( 'NONE',  ( -0.000000000000000000, -0.000000000000000000, 1.000000000000000000 ) ) ;
#59716=ADVANCED_FACE ( 'NONE', ( #61256, #7794, #56316, #8137, #29580, #51049 ), #2859, .T. ) ;
#59736=CARTESIAN_POINT ( 'NONE',  ( -6.000000000000000000, 19.07878402833891229, -20.00000000000000000 ) ) ;
#59783=DIRECTION ( 'NONE',  ( -0.000000000000000000, -0.000000000000000000, 1.000000000000000000 ) ) ;
#59888=AXIS2_PLACEMENT_3D ( 'NONE', #24508, #40661, #7634 ) ;
#59900=DIRECTION ( 'NONE',  ( 1.000000000000000000, 0.000000000000000000, 0.000000000000000000 ) ) ;
#59904=VECTOR ( 'NONE', #5201, 1000.000000000000000 ) ;
#60012=ORIENTED_EDGE ( 'NONE', *, *, #68379, .T. ) ;
#60097=EDGE_CURVE ( 'NONE', #1003, #56426, #9662, .T. ) ;
#60100=DIRECTION ( 'NONE',  ( -0.000000000000000000, -0.000000000000000000, 1.000000000000000000 ) ) ;
#60110=DIRECTION ( 'NONE',  ( -0.000000000000000000, -0.000000000000000000, 1.000000000000000000 ) ) ;
#60346=EDGE_LOOP ( 'NONE', ( #62407, #56124, #49601, #62184 ) ) ;
#60630=AXIS2_PLACEMENT_3D ( 'NONE', #63725, #26437, #58767 ) ;
#60663=CARTESIAN_POINT ( 'NONE',  ( 125.0000000000000000, 1.530808498934191561E-14, -5.000000000000000000 ) ) ;
#60773=CIRCLE ( 'NONE', #50690, 125.0000000000000000 ) ;
#60854=DIRECTION ( 'NONE',  ( 1.000000000000000000, 0.000000000000000000, 0.000000000000000000 ) ) ;
#60905=EDGE_CURVE ( 'NONE', #8320, #15127, #57294, .T. ) ;
#60970=EDGE_LOOP ( 'NONE', ( #46240, #39478, #44759, #67136 ) ) ;
#61014=ADVANCED_FACE ( 'NONE', ( #25213 ), #19571, .F. ) ;
#61016=EDGE_LOOP ( 'NONE', ( #56634, #66277, #16353, #2127 ) ) ;
#61100=DIRECTION ( 'NONE',  ( -0.000000000000000000, -0.000000000000000000, 1.000000000000000000 ) ) ;
#61188=EDGE_CURVE ( 'NONE', #34341, #48842, #17397, .T. ) ;
#61256=FACE_BOUND ( 'NONE', #30617, .T. ) ;
#61573=LINE ( 'NONE', #40801, #30968 ) ;
#61651=VERTEX_POINT ( 'NONE', #50717 ) ;
#61762=FACE_OUTER_BOUND ( 'NONE', #27353, .T. ) ;
#62111=CARTESIAN_POINT ( 'NONE',  ( 0.000000000000000000, 0.000000000000000000, 0.000000000000000000 ) ) ;
#62184=ORIENTED_EDGE ( 'NONE', *, *, #13273, .F. ) ;
#62239=LINE ( 'NONE', #14054, #10651 ) ;
#62264=CARTESIAN_POINT ( 'NONE',  ( 6.000000000000000000, 23.07878402833891229, 9.999999999999998224 ) ) ;
#62407=ORIENTED_EDGE ( 'NONE', *, *, #22852, .T. ) ;
#62435=AXIS2_PLACEMENT_3D ( 'NONE', #40323, #11847, #12555 ) ;
#62487=VECTOR ( 'NONE', #65604, 1000.000000000000000 ) ;
#62494=CONICAL_SURFACE ( 'NONE', #23128, 185.0000000000000000, 1.279339532317029793 ) ;
#62507=CARTESIAN_POINT ( 'NONE',  ( 0.000000000000000000, 0.000000000000000000, 5.000000000000000000 ) ) ;
#62526=CARTESIAN_POINT ( 'NONE',  ( 200.0000000000000000, 0.000000000000000000, 7.000000000000000000 ) ) ;
#62572=CARTESIAN_POINT ( 'NONE',  ( 0.000000000000000000, 0.000000000000000000, 10.00000000000000000 ) ) ;
#62606=CARTESIAN_POINT ( 'NONE',  ( -25.00000000000028066, -65.13282190615278466, -5.000000000000000000 ) ) ;
#62877=FACE_BOUND ( 'NONE', #19110, .T. ) ;
#62891=DIRECTION ( 'NONE',  ( 1.000000000000000000, 0.000000000000000000, 0.000000000000000000 ) ) ;
#62960=DIRECTION ( 'NONE',  ( -0.000000000000000000, -0.000000000000000000, 1.000000000000000000 ) ) ;
#62973=EDGE_CURVE ( 'NONE', #14060, #48814, #4242, .T. ) ;
#63054=FACE_OUTER_BOUND ( 'NONE', #33520, .T. ) ;
#63226=CARTESIAN_POINT ( 'NONE',  ( -200.0000000000000000, 2.449293598294706434E-14, 10.00000000000000000 ) ) ;
#63243=ORIENTED_EDGE ( 'NONE', *, *, #12144, .F. ) ;
#63276=PRODUCT_DEFINITION ( 'UNKNOWN', '', #52341, #73 ) ;
#63317=ORIENTED_EDGE ( 'NONE', *, *, #22852, .F. ) ;
#63351=AXIS2_PLACEMENT_3D ( 'NONE', #9516, #52424, #1034 ) ;
#63433=LINE ( 'NONE', #47923, #52614 ) ;
#63492=ORIENTED_EDGE ( 'NONE', *, *, #48902, .F. ) ;
#63600=EDGE_CURVE ( 'NONE', #30587, #48842, #9908, .T. ) ;
#63695=CIRCLE ( 'NONE', #3053, 25.00000000000145306 ) ;
#63725=CARTESIAN_POINT ( 'NONE',  ( 0.000000000000000000, 0.000000000000000000, -5.000000000000000000 ) ) ;
#63769=DIRECTION ( 'NONE',  ( -1.000000000000000000, 0.000000000000000000, 0.000000000000000000 ) ) ;
#63783=DIRECTION ( 'NONE',  ( -1.000000000000000000, 0.000000000000000000, 0.000000000000000000 ) ) ;
#63869=CARTESIAN_POINT ( 'NONE',  ( 200.0000000000000000, 0.000000000000000000, 10.00000000000000000 ) ) ;
#63979=ORIENTED_EDGE ( 'NONE', *, *, #59128, .F. ) ;
#64047=ORIENTED_EDGE ( 'NONE', *, *, #31698, .T. ) ;
#64257=ORIENTED_EDGE ( 'NONE', *, *, #24805, .T. ) ;
#64281=VERTEX_POINT ( 'NONE', #26405 ) ;
#64384=EDGE_CURVE ( 'NONE', #61651, #14003, #49567, .T. ) ;
#64564=ADVANCED_FACE ( 'NONE', ( #1664 ), #39236, .T. ) ;
#64633=VECTOR ( 'NONE', #29571, 1000.000000000000000 ) ;
#64754=CYLINDRICAL_SURFACE ( 'NONE', #60630, 125.0000000000000000 ) ;
#64798=ADVANCED_FACE ( 'NONE', ( #42062 ), #10055, .T. ) ;
#64810=EDGE_CURVE ( 'NONE', #12453, #48865, #31513, .T. ) ;
#64820=VERTEX_POINT ( 'NONE', #63869 ) ;
#64886=DIRECTION ( 'NONE',  ( -1.000000000000000000, 0.000000000000000000, 0.000000000000000000 ) ) ;
#64951=CARTESIAN_POINT ( 'NONE',  ( -65.13282190615095146, -1.847197903505587038E-12, -9.999999999999998224 ) ) ;
#65023=ORIENTED_EDGE ( 'NONE', *, *, #24558, .F. ) ;
#65125=ORIENTED_EDGE ( 'NONE', *, *, #11570, .F. ) ;
#65199=CARTESIAN_POINT ( 'NONE',  ( 0.000000000000000000, 65.13282190615278466, 5.000000000000000000 ) ) ;
#65202=DIRECTION ( 'NONE',  ( -0.000000000000000000, -0.000000000000000000, 1.000000000000000000 ) ) ;
#65346=CARTESIAN_POINT ( 'NONE',  ( 0.000000000000000000, 0.000000000000000000, -5.000000000000000888 ) ) ;
#65423=ORIENTED_EDGE ( 'NONE', *, *, #30249, .T. ) ;
#65480=DIRECTION ( 'NONE',  ( -0.000000000000000000, -0.000000000000000000, 1.000000000000000000 ) ) ;
#65496=DIRECTION ( 'NONE',  ( 0.000000000000000000, 0.000000000000000000, -1.000000000000000000 ) ) ;
#65604=DIRECTION ( 'NONE',  ( -0.000000000000000000, -0.000000000000000000, -1.000000000000000000 ) ) ;
#65810=ORIENTED_EDGE ( 'NONE', *, *, #63600, .F. ) ;
#65959=ORIENTED_EDGE ( 'NONE', *, *, #6995, .T. ) ;
#65978=EDGE_LOOP ( 'NONE', ( #27225, #48447 ) ) ;
#66123=FACE_OUTER_BOUND ( 'NONE', #60346, .T. ) ;
#66219=AXIS2_PLACEMENT_3D ( 'NONE', #49132, #39305, #38602 ) ;
#66277=ORIENTED_EDGE ( 'NONE', *, *, #44634, .T. ) ;
#66289=EDGE_CURVE ( 'NONE', #66579, #35686, #54923, .T. ) ;
#66299=UNCERTAINTY_MEASURE_WITH_UNIT (LENGTH_MEASURE( 1.000000000000000082E-05 ), #52001, 'distance_accuracy_value', 'NONE');
#66404=CARTESIAN_POINT ( 'NONE',  ( 40.13282190615316836, 1.842283050316774879E-12, 5.000000000000000000 ) ) ;
#66457=DIRECTION ( 'NONE',  ( 1.000000000000000000, 0.000000000000000000, 0.000000000000000000 ) ) ;
#66486=COLOUR_RGB ( '',0.7921568627450980005, 0.8196078431372548767, 0.9333333333333333481 ) ;
#66490=DIRECTION ( 'NONE',  ( 0.000000000000000000, 0.000000000000000000, -1.000000000000000000 ) ) ;
#66567=DIRECTION ( 'NONE',  ( 1.000000000000000000, 0.000000000000000000, 0.000000000000000000 ) ) ;
#66579=VERTEX_POINT ( 'NONE', #68968 ) ;
#66610=DIRECTION ( 'NONE',  ( -0.000000000000000000, -0.000000000000000000, 1.000000000000000000 ) ) ;
#66622=DIRECTION ( 'NONE',  ( 1.000000000000000000, 0.000000000000000000, 0.000000000000000000 ) ) ;
#66690=VERTEX_POINT ( 'NONE', #62606 ) ;
#66742=AXIS2_PLACEMENT_3D ( 'NONE', #33040, #60110, #54831 ) ;
#66793=DIRECTION ( 'NONE',  ( 0.000000000000000000, 0.000000000000000000, -1.000000000000000000 ) ) ;
#66822=EDGE_CURVE ( 'NONE', #64820, #14003, #20454, .T. ) ;
#66832=AXIS2_PLACEMENT_3D ( 'NONE', #50530, #44558, #8319 ) ;
#67012=CIRCLE ( 'NONE', #54571, 25.00000000000000000 ) ;
#67065=CARTESIAN_POINT ( 'NONE',  ( 0.000000000000000000, 0.000000000000000000, -2.500000000000002220 ) ) ;
#67119=CIRCLE ( 'NONE', #17689, 25.00000000000395772 ) ;
#67136=ORIENTED_EDGE ( 'NONE', *, *, #56377, .T. ) ;
#67142=CARTESIAN_POINT ( 'NONE',  ( -65.13282190615095146, -1.847197903505587038E-12, -9.999999999999998224 ) ) ;
#67159=ORIENTED_EDGE ( 'NONE', *, *, #49221, .F. ) ;
#67196=ORIENTED_EDGE ( 'NONE', *, *, #29771, .T. ) ;
#67522=AXIS2_PLACEMENT_3D ( 'NONE', #11419, #32890, #54327 ) ;
#67692=EDGE_LOOP ( 'NONE', ( #43059, #17649, #55407, #36117 ) ) ;
#67832=DIRECTION ( 'NONE',  ( -1.000000000000000000, 0.000000000000000000, 0.000000000000000000 ) ) ;
#67917=DIRECTION ( 'NONE',  ( -1.000000000000000000, 0.000000000000000000, 0.000000000000000000 ) ) ;
#67936=EDGE_CURVE ( 'NONE', #15508, #50826, #5588, .T. ) ;
#68017=AXIS2_PLACEMENT_3D ( 'NONE', #40484, #20076, #31328 ) ;
#68032=EDGE_LOOP ( 'NONE', ( #46638, #18483 ) ) ;
#68141=EDGE_CURVE ( 'NONE', #29280, #16199, #14004, .T. ) ;
#68179=EDGE_LOOP ( 'NONE', ( #14160, #21390, #13252, #45221 ) ) ;
#68301=AXIS2_PLACEMENT_3D ( 'NONE', #26896, #11754, #64886 ) ;
#68379=EDGE_CURVE ( 'NONE', #54841, #383, #16129, .T. ) ;
#68488=DIRECTION ( 'NONE',  ( 0.000000000000000000, -1.000000000000000000, 0.000000000000000000 ) ) ;
#68608=AXIS2_PLACEMENT_3D ( 'NONE', #62111, #3381, #23463 ) ;
#68647=CARTESIAN_POINT ( 'NONE',  ( 0.000000000000000000, 0.000000000000000000, 5.000000000000000000 ) ) ;
#68725=CARTESIAN_POINT ( 'NONE',  ( 0.000000000000000000, 0.000000000000000000, 5.000000000000000000 ) ) ;
#68739=EDGE_LOOP ( 'NONE', ( #20681, #58099, #9514, #59150 ) ) ;
#68968=CARTESIAN_POINT ( 'NONE',  ( 185.0000000000000000, 0.000000000000000000, 2.499999999999999556 ) ) ;
#68976=EDGE_CURVE ( 'NONE', #48814, #14060, #4980, .T. ) ;
#69042=DIRECTION ( 'NONE',  ( 0.000000000000000000, 0.000000000000000000, 1.000000000000000000 ) ) ;
#69142=CARTESIAN_POINT ( 'NONE',  ( -25.00000000000000000, 65.13282190615278466, 5.000000000000000000 ) ) ;
#69393=CARTESIAN_POINT ( 'NONE',  ( -90.13282190615392153, -1.844136286507718230E-12, -9.999999999999998224 ) ) ;
#69540=CARTESIAN_POINT ( 'NONE',  ( -40.13282190614798850, -1.847197903505587038E-12, 5.000000000000000000 ) ) ;
ENDSEC;
END-ISO-10303-21;
